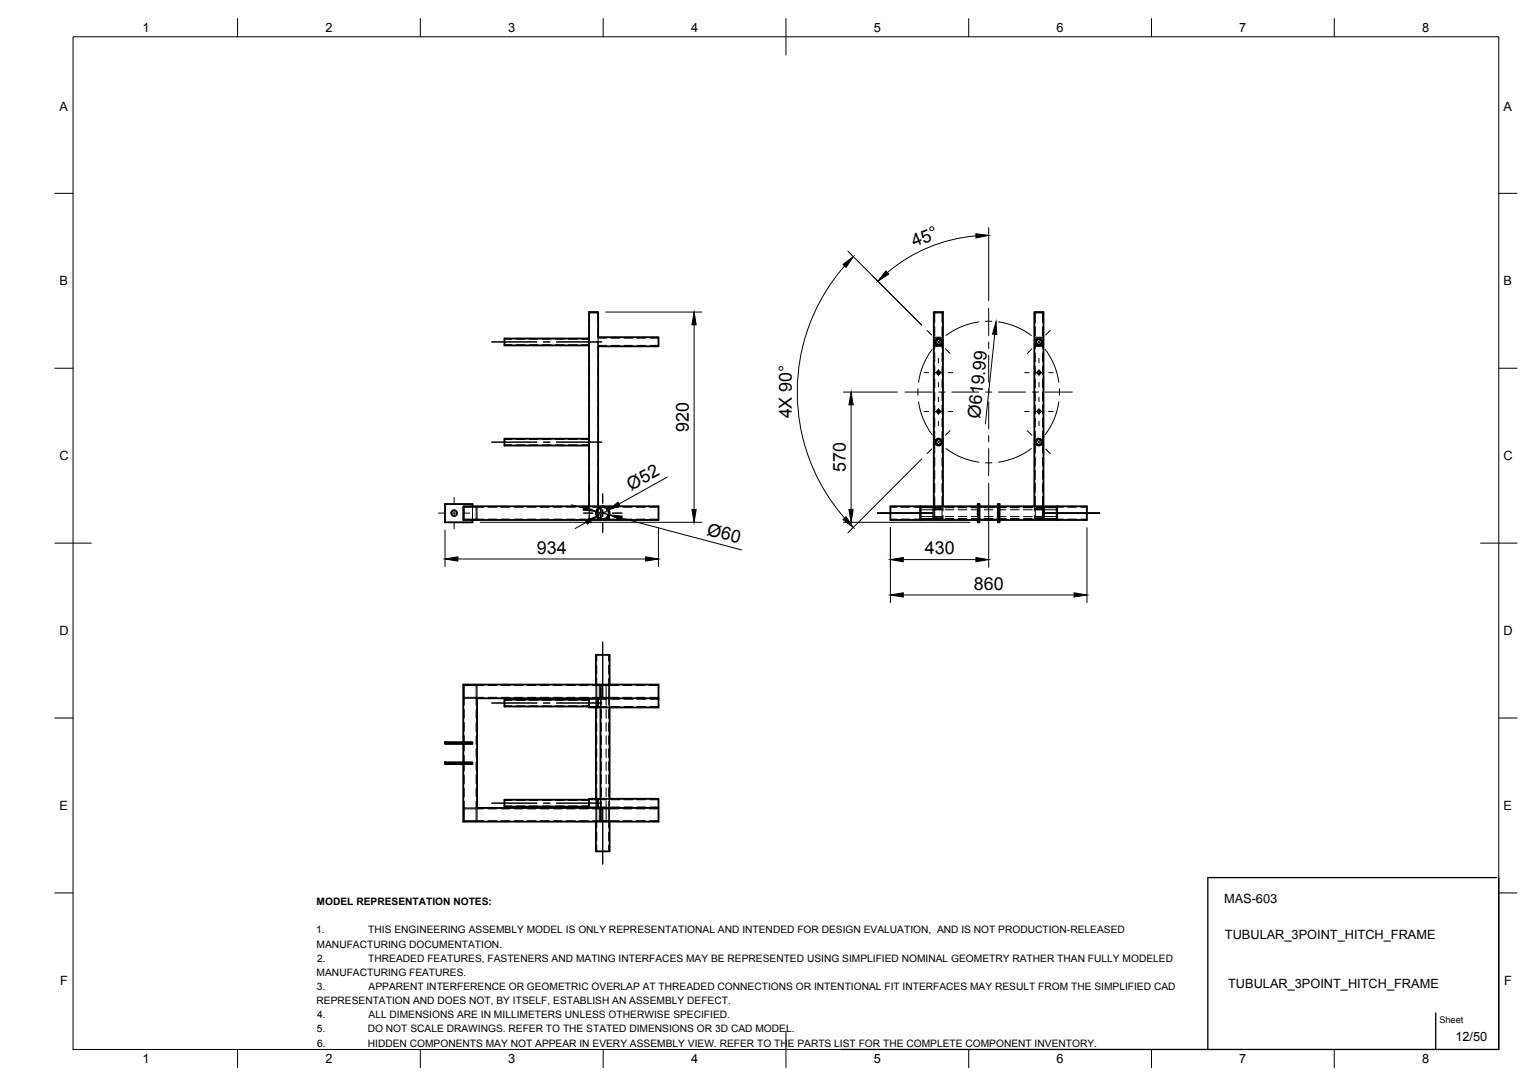
ISO-10303-21;
HEADER;
FILE_DESCRIPTION((''),'2;1');
FILE_NAME('TUBULAR_3POINT_HITCH_FRAME.step','2026-10-01T22:06:14-07:00',(''),(''),'','','');
FILE_SCHEMA (('AUTOMOTIVE_DESIGN { 1 0 10303 214 3 1 1 }'));
ENDSEC;
DATA;
#10=MECHANICAL_DESIGN_GEOMETRIC_PRESENTATION_REPRESENTATION('',(#986),#50440);
#49=ORIENTED_CLOSED_SHELL('',*,#28635,.F.) ;
#50=ORIENTED_CLOSED_SHELL('',*,#28636,.F.) ;
#51=ORIENTED_CLOSED_SHELL('',*,#28637,.F.) ;
#52=ORIENTED_CLOSED_SHELL('',*,#28638,.F.) ;
#53=ORIENTED_CLOSED_SHELL('',*,#28639,.F.) ;
#54=ORIENTED_CLOSED_SHELL('',*,#28640,.F.) ;
#55=ORIENTED_CLOSED_SHELL('',*,#28641,.F.) ;
#56=ORIENTED_CLOSED_SHELL('',*,#28642,.F.) ;
#57=ORIENTED_CLOSED_SHELL('',*,#28643,.F.) ;
#58=ORIENTED_CLOSED_SHELL('',*,#28644,.F.) ;
#59=ORIENTED_CLOSED_SHELL('',*,#28645,.F.) ;
#60=ORIENTED_CLOSED_SHELL('',*,#28646,.F.) ;
#61=ORIENTED_CLOSED_SHELL('',*,#28647,.F.) ;
#62=ORIENTED_CLOSED_SHELL('',*,#28648,.F.) ;
#63=ORIENTED_CLOSED_SHELL('',*,#28649,.F.) ;
#64=ORIENTED_CLOSED_SHELL('',*,#28650,.F.) ;
#65=ORIENTED_CLOSED_SHELL('',*,#28651,.F.) ;
#66=ORIENTED_CLOSED_SHELL('',*,#28652,.F.) ;
#67=ORIENTED_CLOSED_SHELL('',*,#28653,.F.) ;
#79=BREP_WITH_VOIDS('TUBULAR_3POINT_HITCH_FRAME',#28634,(#49,#50,#51,#52,
#53,#54,#55,#56,#57,#58,#59,#60,#61,#62,#63,#64,#65,#66,#67)) ;
#896=SHAPE_REPRESENTATION_RELATIONSHIP('SRR','None',#50627,#941) ;
#941=ADVANCED_BREP_SHAPE_REPRESENTATION('',(#79),#50396) ;
#986=STYLED_ITEM('',(#50883),#79) ;
#1234=FACE_BOUND('',#4462,.T.) ;
#1235=FACE_BOUND('',#4463,.T.) ;
#1236=FACE_BOUND('',#4465,.T.) ;
#1237=FACE_BOUND('',#4466,.T.) ;
#1238=FACE_BOUND('',#4476,.T.) ;
#1239=FACE_BOUND('',#4477,.T.) ;
#1240=FACE_BOUND('',#4479,.T.) ;
#1241=FACE_BOUND('',#4480,.T.) ;
#1242=FACE_BOUND('',#4488,.T.) ;
#1243=FACE_BOUND('',#4490,.T.) ;
#1244=FACE_BOUND('',#4491,.T.) ;
#1245=FACE_BOUND('',#4492,.T.) ;
#1246=FACE_BOUND('',#4493,.T.) ;
#1247=FACE_BOUND('',#4497,.T.) ;
#1248=FACE_BOUND('',#4504,.T.) ;
#1249=FACE_BOUND('',#4508,.T.) ;
#1250=FACE_BOUND('',#4509,.T.) ;
#1251=FACE_BOUND('',#4527,.T.) ;
#1252=FACE_BOUND('',#4536,.T.) ;
#1253=FACE_BOUND('',#4541,.T.) ;
#1254=FACE_BOUND('',#4550,.T.) ;
#1255=FACE_BOUND('',#4552,.T.) ;
#1256=FACE_BOUND('',#4564,.T.) ;
#1257=FACE_BOUND('',#4566,.T.) ;
#1258=FACE_BOUND('',#4569,.T.) ;
#1259=FACE_BOUND('',#4570,.T.) ;
#1260=FACE_BOUND('',#4574,.T.) ;
#1261=FACE_BOUND('',#4581,.T.) ;
#1262=FACE_BOUND('',#4585,.T.) ;
#1263=FACE_BOUND('',#4586,.T.) ;
#1264=FACE_BOUND('',#4587,.T.) ;
#1265=FACE_BOUND('',#4588,.T.) ;
#1266=FACE_BOUND('',#4590,.T.) ;
#1267=FACE_BOUND('',#4605,.T.) ;
#1268=FACE_BOUND('',#4609,.T.) ;
#1269=FACE_BOUND('',#4613,.T.) ;
#1729=PLANE('',#29943) ;
#1730=PLANE('',#29944) ;
#1731=PLANE('',#29945) ;
#1732=PLANE('',#29946) ;
#1733=PLANE('',#29947) ;
#1734=PLANE('',#29948) ;
#1735=PLANE('',#29949) ;
#1736=PLANE('',#29959) ;
#1737=PLANE('',#29960) ;
#1738=PLANE('',#29961) ;
#1739=PLANE('',#29962) ;
#1740=PLANE('',#29963) ;
#1741=PLANE('',#29964) ;
#1742=PLANE('',#29965) ;
#1743=PLANE('',#29978) ;
#1744=PLANE('',#29979) ;
#1745=PLANE('',#29986) ;
#1746=PLANE('',#29987) ;
#1747=PLANE('',#29988) ;
#1748=PLANE('',#29989) ;
#1749=PLANE('',#29990) ;
#1750=PLANE('',#29991) ;
#1751=PLANE('',#29992) ;
#1752=PLANE('',#29993) ;
#1753=PLANE('',#29994) ;
#1754=PLANE('',#29995) ;
#1755=PLANE('',#29996) ;
#1756=PLANE('',#29997) ;
#1757=PLANE('',#29998) ;
#1758=PLANE('',#30000) ;
#1759=PLANE('',#30001) ;
#1760=PLANE('',#30003) ;
#1761=PLANE('',#30004) ;
#1762=PLANE('',#30005) ;
#1763=PLANE('',#30007) ;
#1764=PLANE('',#30009) ;
#1765=PLANE('',#30010) ;
#1766=PLANE('',#30011) ;
#1767=PLANE('',#30012) ;
#1768=PLANE('',#30013) ;
#1769=PLANE('',#30014) ;
#1770=PLANE('',#30016) ;
#1771=PLANE('',#30018) ;
#1772=PLANE('',#30019) ;
#1773=PLANE('',#30021) ;
#1774=PLANE('',#30022) ;
#1775=PLANE('',#30023) ;
#1776=PLANE('',#30024) ;
#1777=PLANE('',#30025) ;
#1778=PLANE('',#30026) ;
#1779=PLANE('',#30027) ;
#1780=PLANE('',#30028) ;
#1781=PLANE('',#30029) ;
#1782=PLANE('',#30031) ;
#1783=PLANE('',#30033) ;
#1784=PLANE('',#30034) ;
#1785=PLANE('',#30035) ;
#1786=PLANE('',#30036) ;
#1787=PLANE('',#30038) ;
#1788=PLANE('',#30039) ;
#1789=PLANE('',#30040) ;
#1790=PLANE('',#30041) ;
#1791=PLANE('',#30042) ;
#1792=PLANE('',#30045) ;
#1793=PLANE('',#30052) ;
#1794=PLANE('',#30053) ;
#1795=PLANE('',#30054) ;
#1796=PLANE('',#30055) ;
#1797=PLANE('',#30056) ;
#1798=PLANE('',#30057) ;
#1799=PLANE('',#30058) ;
#1800=PLANE('',#30059) ;
#1801=PLANE('',#30060) ;
#1802=PLANE('',#30061) ;
#1803=PLANE('',#30062) ;
#1804=PLANE('',#30063) ;
#1805=PLANE('',#30064) ;
#1806=PLANE('',#30065) ;
#1807=PLANE('',#30066) ;
#1808=PLANE('',#30067) ;
#1809=PLANE('',#30068) ;
#1810=PLANE('',#30069) ;
#1811=PLANE('',#30071) ;
#1812=PLANE('',#30077) ;
#1813=PLANE('',#30079) ;
#1814=PLANE('',#30088) ;
#1815=PLANE('',#30089) ;
#1816=PLANE('',#30090) ;
#1817=PLANE('',#30091) ;
#1818=PLANE('',#30092) ;
#1819=PLANE('',#30093) ;
#1820=PLANE('',#30094) ;
#1821=PLANE('',#30095) ;
#1822=PLANE('',#30096) ;
#1823=PLANE('',#30097) ;
#1824=PLANE('',#30098) ;
#1825=PLANE('',#30099) ;
#1826=PLANE('',#30100) ;
#1827=PLANE('',#30101) ;
#1828=PLANE('',#30102) ;
#1829=PLANE('',#30103) ;
#1830=PLANE('',#30104) ;
#1831=PLANE('',#30105) ;
#1832=PLANE('',#30109) ;
#1833=PLANE('',#30110) ;
#1834=PLANE('',#30111) ;
#1835=PLANE('',#30112) ;
#1836=PLANE('',#30113) ;
#1837=PLANE('',#30114) ;
#1838=PLANE('',#30115) ;
#1839=PLANE('',#30117) ;
#1840=PLANE('',#30118) ;
#1841=PLANE('',#30120) ;
#1842=PLANE('',#30122) ;
#1843=PLANE('',#30124) ;
#1844=PLANE('',#30126) ;
#1845=PLANE('',#30128) ;
#1846=PLANE('',#30129) ;
#1847=PLANE('',#30130) ;
#1848=PLANE('',#30132) ;
#1849=PLANE('',#30135) ;
#1850=PLANE('',#30137) ;
#1851=PLANE('',#30138) ;
#1852=PLANE('',#30141) ;
#1853=PLANE('',#30142) ;
#1854=PLANE('',#30143) ;
#1855=PLANE('',#30144) ;
#1856=PLANE('',#30146) ;
#1857=PLANE('',#30149) ;
#1858=PLANE('',#30151) ;
#1859=PLANE('',#30154) ;
#1860=PLANE('',#30155) ;
#1861=PLANE('',#30156) ;
#1862=PLANE('',#30160) ;
#1863=PLANE('',#30161) ;
#1864=PLANE('',#30162) ;
#1865=PLANE('',#30163) ;
#1866=PLANE('',#30165) ;
#1867=PLANE('',#30168) ;
#1868=PLANE('',#30169) ;
#1869=PLANE('',#30170) ;
#1870=PLANE('',#30171) ;
#1871=PLANE('',#30173) ;
#1872=PLANE('',#30179) ;
#1873=PLANE('',#30180) ;
#1874=PLANE('',#30181) ;
#1875=PLANE('',#30182) ;
#1876=PLANE('',#30183) ;
#1877=PLANE('',#30185) ;
#1878=PLANE('',#30191) ;
#1879=PLANE('',#30192) ;
#1880=PLANE('',#30193) ;
#1881=PLANE('',#30194) ;
#1882=PLANE('',#30195) ;
#1883=PLANE('',#30199) ;
#1884=PLANE('',#30200) ;
#1885=PLANE('',#30201) ;
#1886=PLANE('',#30202) ;
#1887=PLANE('',#30203) ;
#1888=PLANE('',#30204) ;
#1889=PLANE('',#30205) ;
#1890=PLANE('',#30206) ;
#1891=PLANE('',#30207) ;
#1892=PLANE('',#30208) ;
#1893=PLANE('',#30209) ;
#1894=PLANE('',#30210) ;
#1895=PLANE('',#30211) ;
#1896=PLANE('',#30212) ;
#1897=PLANE('',#30213) ;
#1898=PLANE('',#30214) ;
#1899=PLANE('',#30215) ;
#1900=PLANE('',#30216) ;
#1901=PLANE('',#30217) ;
#1902=PLANE('',#30218) ;
#1903=PLANE('',#30219) ;
#1904=PLANE('',#30220) ;
#1905=PLANE('',#30221) ;
#1906=PLANE('',#30222) ;
#1907=PLANE('',#30223) ;
#1908=PLANE('',#30224) ;
#1909=PLANE('',#30225) ;
#1910=PLANE('',#30229) ;
#1911=PLANE('',#30230) ;
#1912=PLANE('',#30231) ;
#1913=PLANE('',#30232) ;
#1914=PLANE('',#30234) ;
#1915=PLANE('',#30241) ;
#1916=PLANE('',#30242) ;
#1917=PLANE('',#30243) ;
#1918=PLANE('',#30244) ;
#1919=PLANE('',#30245) ;
#2775=FACE_OUTER_BOUND('',#4451,.T.) ;
#2776=FACE_OUTER_BOUND('',#4452,.T.) ;
#2777=FACE_OUTER_BOUND('',#4453,.T.) ;
#2778=FACE_OUTER_BOUND('',#4454,.T.) ;
#2779=FACE_OUTER_BOUND('',#4455,.T.) ;
#2780=FACE_OUTER_BOUND('',#4456,.T.) ;
#2781=FACE_OUTER_BOUND('',#4457,.T.) ;
#2782=FACE_OUTER_BOUND('',#4458,.T.) ;
#2783=FACE_OUTER_BOUND('',#4459,.T.) ;
#2784=FACE_OUTER_BOUND('',#4460,.T.) ;
#2785=FACE_OUTER_BOUND('',#4461,.T.) ;
#2786=FACE_OUTER_BOUND('',#4464,.T.) ;
#2787=FACE_OUTER_BOUND('',#4467,.T.) ;
#2788=FACE_OUTER_BOUND('',#4468,.T.) ;
#2789=FACE_OUTER_BOUND('',#4469,.T.) ;
#2790=FACE_OUTER_BOUND('',#4470,.T.) ;
#2791=FACE_OUTER_BOUND('',#4471,.T.) ;
#2792=FACE_OUTER_BOUND('',#4472,.T.) ;
#2793=FACE_OUTER_BOUND('',#4473,.T.) ;
#2794=FACE_OUTER_BOUND('',#4474,.T.) ;
#2795=FACE_OUTER_BOUND('',#4475,.T.) ;
#2796=FACE_OUTER_BOUND('',#4478,.T.) ;
#2797=FACE_OUTER_BOUND('',#4481,.T.) ;
#2798=FACE_OUTER_BOUND('',#4482,.T.) ;
#2799=FACE_OUTER_BOUND('',#4483,.T.) ;
#2800=FACE_OUTER_BOUND('',#4484,.T.) ;
#2801=FACE_OUTER_BOUND('',#4485,.T.) ;
#2802=FACE_OUTER_BOUND('',#4486,.T.) ;
#2803=FACE_OUTER_BOUND('',#4487,.T.) ;
#2804=FACE_OUTER_BOUND('',#4489,.T.) ;
#2805=FACE_OUTER_BOUND('',#4494,.T.) ;
#2806=FACE_OUTER_BOUND('',#4495,.T.) ;
#2807=FACE_OUTER_BOUND('',#4496,.T.) ;
#2808=FACE_OUTER_BOUND('',#4498,.T.) ;
#2809=FACE_OUTER_BOUND('',#4499,.T.) ;
#2810=FACE_OUTER_BOUND('',#4500,.T.) ;
#2811=FACE_OUTER_BOUND('',#4501,.T.) ;
#2812=FACE_OUTER_BOUND('',#4502,.T.) ;
#2813=FACE_OUTER_BOUND('',#4503,.T.) ;
#2814=FACE_OUTER_BOUND('',#4505,.T.) ;
#2815=FACE_OUTER_BOUND('',#4506,.T.) ;
#2816=FACE_OUTER_BOUND('',#4507,.T.) ;
#2817=FACE_OUTER_BOUND('',#4510,.T.) ;
#2818=FACE_OUTER_BOUND('',#4511,.T.) ;
#2819=FACE_OUTER_BOUND('',#4512,.T.) ;
#2820=FACE_OUTER_BOUND('',#4513,.T.) ;
#2821=FACE_OUTER_BOUND('',#4514,.T.) ;
#2822=FACE_OUTER_BOUND('',#4515,.T.) ;
#2823=FACE_OUTER_BOUND('',#4516,.T.) ;
#2824=FACE_OUTER_BOUND('',#4517,.T.) ;
#2825=FACE_OUTER_BOUND('',#4518,.T.) ;
#2826=FACE_OUTER_BOUND('',#4519,.T.) ;
#2827=FACE_OUTER_BOUND('',#4520,.T.) ;
#2828=FACE_OUTER_BOUND('',#4521,.T.) ;
#2829=FACE_OUTER_BOUND('',#4522,.T.) ;
#2830=FACE_OUTER_BOUND('',#4523,.T.) ;
#2831=FACE_OUTER_BOUND('',#4524,.T.) ;
#2832=FACE_OUTER_BOUND('',#4525,.T.) ;
#2833=FACE_OUTER_BOUND('',#4526,.T.) ;
#2834=FACE_OUTER_BOUND('',#4528,.T.) ;
#2835=FACE_OUTER_BOUND('',#4529,.T.) ;
#2836=FACE_OUTER_BOUND('',#4530,.T.) ;
#2837=FACE_OUTER_BOUND('',#4531,.T.) ;
#2838=FACE_OUTER_BOUND('',#4532,.T.) ;
#2839=FACE_OUTER_BOUND('',#4533,.T.) ;
#2840=FACE_OUTER_BOUND('',#4534,.T.) ;
#2841=FACE_OUTER_BOUND('',#4535,.T.) ;
#2842=FACE_OUTER_BOUND('',#4537,.T.) ;
#2843=FACE_OUTER_BOUND('',#4538,.T.) ;
#2844=FACE_OUTER_BOUND('',#4539,.T.) ;
#2845=FACE_OUTER_BOUND('',#4540,.T.) ;
#2846=FACE_OUTER_BOUND('',#4542,.T.) ;
#2847=FACE_OUTER_BOUND('',#4543,.T.) ;
#2848=FACE_OUTER_BOUND('',#4544,.T.) ;
#2849=FACE_OUTER_BOUND('',#4545,.T.) ;
#2850=FACE_OUTER_BOUND('',#4546,.T.) ;
#2851=FACE_OUTER_BOUND('',#4547,.T.) ;
#2852=FACE_OUTER_BOUND('',#4548,.T.) ;
#2853=FACE_OUTER_BOUND('',#4549,.T.) ;
#2854=FACE_OUTER_BOUND('',#4551,.T.) ;
#2855=FACE_OUTER_BOUND('',#4553,.T.) ;
#2856=FACE_OUTER_BOUND('',#4554,.T.) ;
#2857=FACE_OUTER_BOUND('',#4555,.T.) ;
#2858=FACE_OUTER_BOUND('',#4556,.T.) ;
#2859=FACE_OUTER_BOUND('',#4557,.T.) ;
#2860=FACE_OUTER_BOUND('',#4558,.T.) ;
#2861=FACE_OUTER_BOUND('',#4559,.T.) ;
#2862=FACE_OUTER_BOUND('',#4560,.T.) ;
#2863=FACE_OUTER_BOUND('',#4561,.T.) ;
#2864=FACE_OUTER_BOUND('',#4562,.T.) ;
#2865=FACE_OUTER_BOUND('',#4563,.T.) ;
#2866=FACE_OUTER_BOUND('',#4565,.T.) ;
#2867=FACE_OUTER_BOUND('',#4567,.T.) ;
#2868=FACE_OUTER_BOUND('',#4568,.T.) ;
#2869=FACE_OUTER_BOUND('',#4571,.T.) ;
#2870=FACE_OUTER_BOUND('',#4572,.T.) ;
#2871=FACE_OUTER_BOUND('',#4573,.T.) ;
#2872=FACE_OUTER_BOUND('',#4575,.T.) ;
#2873=FACE_OUTER_BOUND('',#4576,.T.) ;
#2874=FACE_OUTER_BOUND('',#4577,.T.) ;
#2875=FACE_OUTER_BOUND('',#4578,.T.) ;
#2876=FACE_OUTER_BOUND('',#4579,.T.) ;
#2877=FACE_OUTER_BOUND('',#4580,.T.) ;
#2878=FACE_OUTER_BOUND('',#4582,.T.) ;
#2879=FACE_OUTER_BOUND('',#4583,.T.) ;
#2880=FACE_OUTER_BOUND('',#4584,.T.) ;
#2881=FACE_OUTER_BOUND('',#4589,.T.) ;
#2882=FACE_OUTER_BOUND('',#4591,.T.) ;
#2883=FACE_OUTER_BOUND('',#4592,.T.) ;
#2884=FACE_OUTER_BOUND('',#4593,.T.) ;
#2885=FACE_OUTER_BOUND('',#4594,.T.) ;
#2886=FACE_OUTER_BOUND('',#4595,.T.) ;
#2887=FACE_OUTER_BOUND('',#4596,.T.) ;
#2888=FACE_OUTER_BOUND('',#4597,.T.) ;
#2889=FACE_OUTER_BOUND('',#4598,.T.) ;
#2890=FACE_OUTER_BOUND('',#4599,.T.) ;
#2891=FACE_OUTER_BOUND('',#4600,.T.) ;
#2892=FACE_OUTER_BOUND('',#4601,.T.) ;
#2893=FACE_OUTER_BOUND('',#4602,.T.) ;
#2894=FACE_OUTER_BOUND('',#4603,.T.) ;
#2895=FACE_OUTER_BOUND('',#4604,.T.) ;
#2896=FACE_OUTER_BOUND('',#4606,.T.) ;
#2897=FACE_OUTER_BOUND('',#4607,.T.) ;
#2898=FACE_OUTER_BOUND('',#4608,.T.) ;
#2899=FACE_OUTER_BOUND('',#4610,.T.) ;
#2900=FACE_OUTER_BOUND('',#4611,.T.) ;
#2901=FACE_OUTER_BOUND('',#4612,.T.) ;
#2902=FACE_OUTER_BOUND('',#4614,.T.) ;
#2903=FACE_OUTER_BOUND('',#4615,.T.) ;
#2904=FACE_OUTER_BOUND('',#4616,.T.) ;
#2905=FACE_OUTER_BOUND('',#4617,.T.) ;
#2906=FACE_OUTER_BOUND('',#4618,.T.) ;
#2907=FACE_OUTER_BOUND('',#4619,.T.) ;
#2908=FACE_OUTER_BOUND('',#4620,.T.) ;
#2909=FACE_OUTER_BOUND('',#4621,.T.) ;
#2910=FACE_OUTER_BOUND('',#4622,.T.) ;
#2911=FACE_OUTER_BOUND('',#4623,.T.) ;
#2912=FACE_OUTER_BOUND('',#4624,.T.) ;
#2913=FACE_OUTER_BOUND('',#4625,.T.) ;
#2914=FACE_OUTER_BOUND('',#4626,.T.) ;
#2915=FACE_OUTER_BOUND('',#4627,.T.) ;
#2916=FACE_OUTER_BOUND('',#4628,.T.) ;
#2917=FACE_OUTER_BOUND('',#4629,.T.) ;
#2918=FACE_OUTER_BOUND('',#4630,.T.) ;
#2919=FACE_OUTER_BOUND('',#4631,.T.) ;
#2920=FACE_OUTER_BOUND('',#4632,.T.) ;
#2921=FACE_OUTER_BOUND('',#4633,.T.) ;
#2922=FACE_OUTER_BOUND('',#4634,.T.) ;
#2923=FACE_OUTER_BOUND('',#4635,.T.) ;
#2924=FACE_OUTER_BOUND('',#4636,.T.) ;
#2925=FACE_OUTER_BOUND('',#4637,.T.) ;
#2926=FACE_OUTER_BOUND('',#4638,.T.) ;
#2927=FACE_OUTER_BOUND('',#4639,.T.) ;
#2928=FACE_OUTER_BOUND('',#4640,.T.) ;
#2929=FACE_OUTER_BOUND('',#4641,.T.) ;
#2930=FACE_OUTER_BOUND('',#4642,.T.) ;
#2931=FACE_OUTER_BOUND('',#4643,.T.) ;
#2932=FACE_OUTER_BOUND('',#4644,.T.) ;
#2933=FACE_OUTER_BOUND('',#4645,.T.) ;
#2934=FACE_OUTER_BOUND('',#4646,.T.) ;
#2935=FACE_OUTER_BOUND('',#4647,.T.) ;
#2936=FACE_OUTER_BOUND('',#4648,.T.) ;
#2937=FACE_OUTER_BOUND('',#4649,.T.) ;
#2938=FACE_OUTER_BOUND('',#4650,.T.) ;
#2939=FACE_OUTER_BOUND('',#4651,.T.) ;
#2940=FACE_OUTER_BOUND('',#4652,.T.) ;
#2941=FACE_OUTER_BOUND('',#4653,.T.) ;
#2942=FACE_OUTER_BOUND('',#4654,.T.) ;
#2943=FACE_OUTER_BOUND('',#4655,.T.) ;
#2944=FACE_OUTER_BOUND('',#4656,.T.) ;
#2945=FACE_OUTER_BOUND('',#4657,.T.) ;
#2946=FACE_OUTER_BOUND('',#4658,.T.) ;
#2947=FACE_OUTER_BOUND('',#4659,.T.) ;
#2948=FACE_OUTER_BOUND('',#4660,.T.) ;
#2949=FACE_OUTER_BOUND('',#4661,.T.) ;
#2950=FACE_OUTER_BOUND('',#4662,.T.) ;
#2951=FACE_OUTER_BOUND('',#4663,.T.) ;
#2952=FACE_OUTER_BOUND('',#4664,.T.) ;
#2953=FACE_OUTER_BOUND('',#4665,.T.) ;
#2954=FACE_OUTER_BOUND('',#4666,.T.) ;
#2955=FACE_OUTER_BOUND('',#4667,.T.) ;
#2956=FACE_OUTER_BOUND('',#4668,.T.) ;
#2957=FACE_OUTER_BOUND('',#4669,.T.) ;
#2958=FACE_OUTER_BOUND('',#4670,.T.) ;
#2959=FACE_OUTER_BOUND('',#4671,.T.) ;
#2960=FACE_OUTER_BOUND('',#4672,.T.) ;
#2961=FACE_OUTER_BOUND('',#4673,.T.) ;
#2962=FACE_OUTER_BOUND('',#4674,.T.) ;
#2963=FACE_OUTER_BOUND('',#4675,.T.) ;
#2964=FACE_OUTER_BOUND('',#4676,.T.) ;
#2965=FACE_OUTER_BOUND('',#4677,.T.) ;
#2966=FACE_OUTER_BOUND('',#4678,.T.) ;
#2967=FACE_OUTER_BOUND('',#4679,.T.) ;
#2968=FACE_OUTER_BOUND('',#4680,.T.) ;
#2969=FACE_OUTER_BOUND('',#4681,.T.) ;
#2970=FACE_OUTER_BOUND('',#4682,.T.) ;
#2971=FACE_OUTER_BOUND('',#4683,.T.) ;
#2972=FACE_OUTER_BOUND('',#4684,.T.) ;
#2973=FACE_OUTER_BOUND('',#4685,.T.) ;
#2974=FACE_OUTER_BOUND('',#4686,.T.) ;
#2975=FACE_OUTER_BOUND('',#4687,.T.) ;
#2976=FACE_OUTER_BOUND('',#4688,.T.) ;
#2977=FACE_OUTER_BOUND('',#4689,.T.) ;
#2978=FACE_OUTER_BOUND('',#4690,.T.) ;
#2979=FACE_OUTER_BOUND('',#4691,.T.) ;
#2980=FACE_OUTER_BOUND('',#4692,.T.) ;
#2981=FACE_OUTER_BOUND('',#4693,.T.) ;
#2982=FACE_OUTER_BOUND('',#4694,.T.) ;
#2983=FACE_OUTER_BOUND('',#4695,.T.) ;
#2984=FACE_OUTER_BOUND('',#4696,.T.) ;
#2985=FACE_OUTER_BOUND('',#4697,.T.) ;
#2986=FACE_OUTER_BOUND('',#4698,.T.) ;
#2987=FACE_OUTER_BOUND('',#4699,.T.) ;
#2988=FACE_OUTER_BOUND('',#4700,.T.) ;
#2989=FACE_OUTER_BOUND('',#4701,.T.) ;
#2990=FACE_OUTER_BOUND('',#4702,.T.) ;
#2991=FACE_OUTER_BOUND('',#4703,.T.) ;
#2992=FACE_OUTER_BOUND('',#4704,.T.) ;
#2993=FACE_OUTER_BOUND('',#4705,.T.) ;
#2994=FACE_OUTER_BOUND('',#4706,.T.) ;
#2995=FACE_OUTER_BOUND('',#4707,.T.) ;
#2996=FACE_OUTER_BOUND('',#4708,.T.) ;
#2997=FACE_OUTER_BOUND('',#4709,.T.) ;
#2998=FACE_OUTER_BOUND('',#4710,.T.) ;
#2999=FACE_OUTER_BOUND('',#4711,.T.) ;
#3000=FACE_OUTER_BOUND('',#4712,.T.) ;
#3001=FACE_OUTER_BOUND('',#4713,.T.) ;
#3002=FACE_OUTER_BOUND('',#4714,.T.) ;
#3003=FACE_OUTER_BOUND('',#4715,.T.) ;
#3004=FACE_OUTER_BOUND('',#4716,.T.) ;
#3005=FACE_OUTER_BOUND('',#4717,.T.) ;
#3006=FACE_OUTER_BOUND('',#4718,.T.) ;
#4451=EDGE_LOOP('',(#21063,#21064,#21065,#21066)) ;
#4452=EDGE_LOOP('',(#21067,#21068,#21069,#21070)) ;
#4453=EDGE_LOOP('',(#21071,#21072,#21073,#21074)) ;
#4454=EDGE_LOOP('',(#21075,#21076,#21077,#21078)) ;
#4455=EDGE_LOOP('',(#21079,#21080,#21081,#21082)) ;
#4456=EDGE_LOOP('',(#21083,#21084,#21085,#21086)) ;
#4457=EDGE_LOOP('',(#21087,#21088,#21089,#21090)) ;
#4458=EDGE_LOOP('',(#21091,#21092,#21093,#21094)) ;
#4459=EDGE_LOOP('',(#21095,#21096,#21097,#21098,#21099,#21100)) ;
#4460=EDGE_LOOP('',(#21101,#21102,#21103,#21104)) ;
#4461=EDGE_LOOP('',(#21105,#21106,#21107,#21108)) ;
#4462=EDGE_LOOP('',(#21109)) ;
#4463=EDGE_LOOP('',(#21110)) ;
#4464=EDGE_LOOP('',(#21111,#21112,#21113,#21114)) ;
#4465=EDGE_LOOP('',(#21115)) ;
#4466=EDGE_LOOP('',(#21116)) ;
#4467=EDGE_LOOP('',(#21117,#21118,#21119,#21120)) ;
#4468=EDGE_LOOP('',(#21121,#21122,#21123,#21124,#21125,#21126)) ;
#4469=EDGE_LOOP('',(#21127,#21128,#21129,#21130)) ;
#4470=EDGE_LOOP('',(#21131,#21132,#21133,#21134)) ;
#4471=EDGE_LOOP('',(#21135,#21136,#21137,#21138)) ;
#4472=EDGE_LOOP('',(#21139,#21140,#21141,#21142)) ;
#4473=EDGE_LOOP('',(#21143,#21144,#21145,#21146,#21147,#21148)) ;
#4474=EDGE_LOOP('',(#21149,#21150,#21151,#21152)) ;
#4475=EDGE_LOOP('',(#21153,#21154,#21155,#21156)) ;
#4476=EDGE_LOOP('',(#21157)) ;
#4477=EDGE_LOOP('',(#21158)) ;
#4478=EDGE_LOOP('',(#21159,#21160,#21161,#21162)) ;
#4479=EDGE_LOOP('',(#21163)) ;
#4480=EDGE_LOOP('',(#21164)) ;
#4481=EDGE_LOOP('',(#21165,#21166,#21167,#21168)) ;
#4482=EDGE_LOOP('',(#21169,#21170,#21171,#21172,#21173,#21174)) ;
#4483=EDGE_LOOP('',(#21175,#21176,#21177,#21178)) ;
#4484=EDGE_LOOP('',(#21179,#21180,#21181,#21182)) ;
#4485=EDGE_LOOP('',(#21183,#21184,#21185,#21186)) ;
#4486=EDGE_LOOP('',(#21187,#21188,#21189,#21190)) ;
#4487=EDGE_LOOP('',(#21191)) ;
#4488=EDGE_LOOP('',(#21192)) ;
#4489=EDGE_LOOP('',(#21193,#21194,#21195,#21196,#21197)) ;
#4490=EDGE_LOOP('',(#21198)) ;
#4491=EDGE_LOOP('',(#21199)) ;
#4492=EDGE_LOOP('',(#21200)) ;
#4493=EDGE_LOOP('',(#21201)) ;
#4494=EDGE_LOOP('',(#21202,#21203,#21204,#21205)) ;
#4495=EDGE_LOOP('',(#21206,#21207,#21208,#21209)) ;
#4496=EDGE_LOOP('',(#21210)) ;
#4497=EDGE_LOOP('',(#21211)) ;
#4498=EDGE_LOOP('',(#21212)) ;
#4499=EDGE_LOOP('',(#21213,#21214,#21215,#21216)) ;
#4500=EDGE_LOOP('',(#21217,#21218,#21219,#21220)) ;
#4501=EDGE_LOOP('',(#21221,#21222,#21223,#21224)) ;
#4502=EDGE_LOOP('',(#21225,#21226,#21227,#21228)) ;
#4503=EDGE_LOOP('',(#21229,#21230,#21231,#21232)) ;
#4504=EDGE_LOOP('',(#21233,#21234,#21235,#21236)) ;
#4505=EDGE_LOOP('',(#21237,#21238,#21239,#21240)) ;
#4506=EDGE_LOOP('',(#21241,#21242,#21243,#21244)) ;
#4507=EDGE_LOOP('',(#21245,#21246,#21247,#21248,#21249)) ;
#4508=EDGE_LOOP('',(#21250)) ;
#4509=EDGE_LOOP('',(#21251)) ;
#4510=EDGE_LOOP('',(#21252,#21253,#21254,#21255)) ;
#4511=EDGE_LOOP('',(#21256,#21257,#21258,#21259)) ;
#4512=EDGE_LOOP('',(#21260)) ;
#4513=EDGE_LOOP('',(#21261,#21262,#21263,#21264)) ;
#4514=EDGE_LOOP('',(#21265,#21266,#21267,#21268,#21269,#21270,#21271,#21272,
#21273,#21274)) ;
#4515=EDGE_LOOP('',(#21275,#21276,#21277,#21278,#21279,#21280,#21281,#21282)) ;
#4516=EDGE_LOOP('',(#21283,#21284,#21285,#21286)) ;
#4517=EDGE_LOOP('',(#21287,#21288,#21289,#21290)) ;
#4518=EDGE_LOOP('',(#21291,#21292,#21293,#21294)) ;
#4519=EDGE_LOOP('',(#21295,#21296,#21297,#21298)) ;
#4520=EDGE_LOOP('',(#21299,#21300,#21301,#21302)) ;
#4521=EDGE_LOOP('',(#21303,#21304,#21305,#21306)) ;
#4522=EDGE_LOOP('',(#21307,#21308,#21309,#21310)) ;
#4523=EDGE_LOOP('',(#21311,#21312,#21313,#21314)) ;
#4524=EDGE_LOOP('',(#21315,#21316,#21317,#21318)) ;
#4525=EDGE_LOOP('',(#21319,#21320,#21321,#21322)) ;
#4526=EDGE_LOOP('',(#21323,#21324,#21325,#21326,#21327,#21328,#21329,#21330,
#21331,#21332,#21333,#21334,#21335,#21336,#21337,#21338,#21339,#21340)) ;
#4527=EDGE_LOOP('',(#21341,#21342,#21343,#21344,#21345,#21346,#21347,#21348,
#21349,#21350,#21351,#21352)) ;
#4528=EDGE_LOOP('',(#21353,#21354,#21355,#21356)) ;
#4529=EDGE_LOOP('',(#21357,#21358,#21359,#21360)) ;
#4530=EDGE_LOOP('',(#21361,#21362,#21363,#21364)) ;
#4531=EDGE_LOOP('',(#21365,#21366,#21367,#21368)) ;
#4532=EDGE_LOOP('',(#21369,#21370,#21371,#21372)) ;
#4533=EDGE_LOOP('',(#21373,#21374,#21375,#21376)) ;
#4534=EDGE_LOOP('',(#21377,#21378,#21379,#21380)) ;
#4535=EDGE_LOOP('',(#21381,#21382,#21383,#21384)) ;
#4536=EDGE_LOOP('',(#21385,#21386,#21387,#21388)) ;
#4537=EDGE_LOOP('',(#21389,#21390,#21391,#21392)) ;
#4538=EDGE_LOOP('',(#21393)) ;
#4539=EDGE_LOOP('',(#21394)) ;
#4540=EDGE_LOOP('',(#21395,#21396,#21397,#21398)) ;
#4541=EDGE_LOOP('',(#21399,#21400,#21401,#21402)) ;
#4542=EDGE_LOOP('',(#21403,#21404,#21405,#21406)) ;
#4543=EDGE_LOOP('',(#21407,#21408,#21409,#21410)) ;
#4544=EDGE_LOOP('',(#21411,#21412,#21413,#21414)) ;
#4545=EDGE_LOOP('',(#21415,#21416,#21417,#21418)) ;
#4546=EDGE_LOOP('',(#21419,#21420,#21421,#21422)) ;
#4547=EDGE_LOOP('',(#21423,#21424,#21425,#21426)) ;
#4548=EDGE_LOOP('',(#21427,#21428,#21429,#21430)) ;
#4549=EDGE_LOOP('',(#21431)) ;
#4550=EDGE_LOOP('',(#21432)) ;
#4551=EDGE_LOOP('',(#21433)) ;
#4552=EDGE_LOOP('',(#21434)) ;
#4553=EDGE_LOOP('',(#21435,#21436,#21437,#21438,#21439)) ;
#4554=EDGE_LOOP('',(#21440,#21441,#21442,#21443,#21444)) ;
#4555=EDGE_LOOP('',(#21445,#21446,#21447,#21448)) ;
#4556=EDGE_LOOP('',(#21449,#21450,#21451,#21452)) ;
#4557=EDGE_LOOP('',(#21453,#21454,#21455,#21456)) ;
#4558=EDGE_LOOP('',(#21457,#21458,#21459,#21460)) ;
#4559=EDGE_LOOP('',(#21461,#21462,#21463,#21464)) ;
#4560=EDGE_LOOP('',(#21465,#21466,#21467,#21468)) ;
#4561=EDGE_LOOP('',(#21469,#21470,#21471,#21472)) ;
#4562=EDGE_LOOP('',(#21473,#21474,#21475,#21476)) ;
#4563=EDGE_LOOP('',(#21477,#21478,#21479,#21480,#21481,#21482,#21483,#21484)) ;
#4564=EDGE_LOOP('',(#21485)) ;
#4565=EDGE_LOOP('',(#21486,#21487,#21488,#21489,#21490,#21491,#21492,#21493)) ;
#4566=EDGE_LOOP('',(#21494)) ;
#4567=EDGE_LOOP('',(#21495,#21496,#21497,#21498)) ;
#4568=EDGE_LOOP('',(#21499,#21500,#21501,#21502,#21503)) ;
#4569=EDGE_LOOP('',(#21504)) ;
#4570=EDGE_LOOP('',(#21505)) ;
#4571=EDGE_LOOP('',(#21506,#21507,#21508,#21509)) ;
#4572=EDGE_LOOP('',(#21510,#21511,#21512,#21513)) ;
#4573=EDGE_LOOP('',(#21514,#21515,#21516,#21517)) ;
#4574=EDGE_LOOP('',(#21518,#21519,#21520,#21521)) ;
#4575=EDGE_LOOP('',(#21522,#21523,#21524,#21525)) ;
#4576=EDGE_LOOP('',(#21526,#21527,#21528,#21529)) ;
#4577=EDGE_LOOP('',(#21530,#21531,#21532,#21533)) ;
#4578=EDGE_LOOP('',(#21534,#21535,#21536,#21537)) ;
#4579=EDGE_LOOP('',(#21538)) ;
#4580=EDGE_LOOP('',(#21539)) ;
#4581=EDGE_LOOP('',(#21540)) ;
#4582=EDGE_LOOP('',(#21541,#21542,#21543,#21544)) ;
#4583=EDGE_LOOP('',(#21545,#21546,#21547,#21548)) ;
#4584=EDGE_LOOP('',(#21549,#21550,#21551,#21552,#21553)) ;
#4585=EDGE_LOOP('',(#21554)) ;
#4586=EDGE_LOOP('',(#21555)) ;
#4587=EDGE_LOOP('',(#21556)) ;
#4588=EDGE_LOOP('',(#21557)) ;
#4589=EDGE_LOOP('',(#21558)) ;
#4590=EDGE_LOOP('',(#21559)) ;
#4591=EDGE_LOOP('',(#21560,#21561,#21562,#21563)) ;
#4592=EDGE_LOOP('',(#21564,#21565,#21566,#21567)) ;
#4593=EDGE_LOOP('',(#21568,#21569,#21570,#21571,#21572,#21573,#21574,#21575,
#21576,#21577,#21578,#21579)) ;
#4594=EDGE_LOOP('',(#21580,#21581,#21582,#21583)) ;
#4595=EDGE_LOOP('',(#21584,#21585,#21586,#21587)) ;
#4596=EDGE_LOOP('',(#21588,#21589,#21590,#21591)) ;
#4597=EDGE_LOOP('',(#21592,#21593,#21594,#21595)) ;
#4598=EDGE_LOOP('',(#21596,#21597,#21598,#21599,#21600,#21601,#21602,#21603,
#21604,#21605)) ;
#4599=EDGE_LOOP('',(#21606)) ;
#4600=EDGE_LOOP('',(#21607,#21608,#21609,#21610)) ;
#4601=EDGE_LOOP('',(#21611,#21612,#21613,#21614)) ;
#4602=EDGE_LOOP('',(#21615,#21616,#21617,#21618,#21619,#21620,#21621,#21622)) ;
#4603=EDGE_LOOP('',(#21623,#21624,#21625,#21626)) ;
#4604=EDGE_LOOP('',(#21627,#21628,#21629,#21630,#21631,#21632,#21633,#21634,
#21635,#21636,#21637,#21638,#21639,#21640,#21641,#21642,#21643,#21644)) ;
#4605=EDGE_LOOP('',(#21645,#21646,#21647,#21648,#21649,#21650,#21651,#21652)) ;
#4606=EDGE_LOOP('',(#21653,#21654,#21655,#21656)) ;
#4607=EDGE_LOOP('',(#21657,#21658,#21659,#21660)) ;
#4608=EDGE_LOOP('',(#21661,#21662,#21663,#21664,#21665,#21666,#21667,#21668)) ;
#4609=EDGE_LOOP('',(#21669)) ;
#4610=EDGE_LOOP('',(#21670,#21671,#21672,#21673)) ;
#4611=EDGE_LOOP('',(#21674,#21675,#21676,#21677)) ;
#4612=EDGE_LOOP('',(#21678,#21679,#21680,#21681,#21682,#21683,#21684,#21685)) ;
#4613=EDGE_LOOP('',(#21686)) ;
#4614=EDGE_LOOP('',(#21687,#21688,#21689,#21690)) ;
#4615=EDGE_LOOP('',(#21691,#21692,#21693,#21694)) ;
#4616=EDGE_LOOP('',(#21695,#21696,#21697,#21698)) ;
#4617=EDGE_LOOP('',(#21699,#21700,#21701,#21702)) ;
#4618=EDGE_LOOP('',(#21703,#21704,#21705,#21706)) ;
#4619=EDGE_LOOP('',(#21707,#21708,#21709,#21710)) ;
#4620=EDGE_LOOP('',(#21711,#21712,#21713,#21714)) ;
#4621=EDGE_LOOP('',(#21715,#21716,#21717,#21718)) ;
#4622=EDGE_LOOP('',(#21719,#21720,#21721,#21722)) ;
#4623=EDGE_LOOP('',(#21723,#21724,#21725,#21726)) ;
#4624=EDGE_LOOP('',(#21727,#21728,#21729,#21730)) ;
#4625=EDGE_LOOP('',(#21731,#21732,#21733,#21734)) ;
#4626=EDGE_LOOP('',(#21735,#21736,#21737,#21738)) ;
#4627=EDGE_LOOP('',(#21739,#21740)) ;
#4628=EDGE_LOOP('',(#21741,#21742)) ;
#4629=EDGE_LOOP('',(#21743,#21744,#21745,#21746)) ;
#4630=EDGE_LOOP('',(#21747,#21748,#21749,#21750)) ;
#4631=EDGE_LOOP('',(#21751,#21752,#21753,#21754)) ;
#4632=EDGE_LOOP('',(#21755,#21756,#21757,#21758)) ;
#4633=EDGE_LOOP('',(#21759,#21760,#21761)) ;
#4634=EDGE_LOOP('',(#21762,#21763,#21764)) ;
#4635=EDGE_LOOP('',(#21765,#21766,#21767,#21768)) ;
#4636=EDGE_LOOP('',(#21769,#21770,#21771)) ;
#4637=EDGE_LOOP('',(#21772,#21773,#21774,#21775)) ;
#4638=EDGE_LOOP('',(#21776,#21777,#21778)) ;
#4639=EDGE_LOOP('',(#21779,#21780,#21781,#21782)) ;
#4640=EDGE_LOOP('',(#21783,#21784,#21785,#21786)) ;
#4641=EDGE_LOOP('',(#21787,#21788,#21789,#21790)) ;
#4642=EDGE_LOOP('',(#21791,#21792,#21793,#21794)) ;
#4643=EDGE_LOOP('',(#21795,#21796,#21797)) ;
#4644=EDGE_LOOP('',(#21798,#21799,#21800)) ;
#4645=EDGE_LOOP('',(#21801,#21802,#21803,#21804)) ;
#4646=EDGE_LOOP('',(#21805,#21806,#21807)) ;
#4647=EDGE_LOOP('',(#21808,#21809,#21810)) ;
#4648=EDGE_LOOP('',(#21811,#21812,#21813,#21814)) ;
#4649=EDGE_LOOP('',(#21815,#21816,#21817,#21818)) ;
#4650=EDGE_LOOP('',(#21819,#21820,#21821,#21822)) ;
#4651=EDGE_LOOP('',(#21823,#21824,#21825,#21826)) ;
#4652=EDGE_LOOP('',(#21827,#21828,#21829,#21830)) ;
#4653=EDGE_LOOP('',(#21831,#21832,#21833)) ;
#4654=EDGE_LOOP('',(#21834,#21835,#21836,#21837)) ;
#4655=EDGE_LOOP('',(#21838,#21839,#21840)) ;
#4656=EDGE_LOOP('',(#21841,#21842,#21843)) ;
#4657=EDGE_LOOP('',(#21844,#21845,#21846)) ;
#4658=EDGE_LOOP('',(#21847,#21848,#21849,#21850)) ;
#4659=EDGE_LOOP('',(#21851,#21852,#21853,#21854)) ;
#4660=EDGE_LOOP('',(#21855,#21856,#21857,#21858)) ;
#4661=EDGE_LOOP('',(#21859,#21860,#21861,#21862)) ;
#4662=EDGE_LOOP('',(#21863,#21864)) ;
#4663=EDGE_LOOP('',(#21865,#21866)) ;
#4664=EDGE_LOOP('',(#21867,#21868,#21869,#21870)) ;
#4665=EDGE_LOOP('',(#21871,#21872,#21873,#21874)) ;
#4666=EDGE_LOOP('',(#21875,#21876)) ;
#4667=EDGE_LOOP('',(#21877,#21878)) ;
#4668=EDGE_LOOP('',(#21879,#21880,#21881,#21882)) ;
#4669=EDGE_LOOP('',(#21883,#21884,#21885,#21886)) ;
#4670=EDGE_LOOP('',(#21887,#21888)) ;
#4671=EDGE_LOOP('',(#21889,#21890)) ;
#4672=EDGE_LOOP('',(#21891,#21892,#21893,#21894)) ;
#4673=EDGE_LOOP('',(#21895,#21896,#21897,#21898)) ;
#4674=EDGE_LOOP('',(#21899,#21900)) ;
#4675=EDGE_LOOP('',(#21901,#21902)) ;
#4676=EDGE_LOOP('',(#21903,#21904,#21905,#21906)) ;
#4677=EDGE_LOOP('',(#21907,#21908,#21909,#21910)) ;
#4678=EDGE_LOOP('',(#21911,#21912)) ;
#4679=EDGE_LOOP('',(#21913,#21914,#21915,#21916)) ;
#4680=EDGE_LOOP('',(#21917,#21918)) ;
#4681=EDGE_LOOP('',(#21919,#21920,#21921,#21922)) ;
#4682=EDGE_LOOP('',(#21923,#21924,#21925,#21926)) ;
#4683=EDGE_LOOP('',(#21927,#21928,#21929,#21930)) ;
#4684=EDGE_LOOP('',(#21931,#21932,#21933,#21934)) ;
#4685=EDGE_LOOP('',(#21935,#21936,#21937,#21938)) ;
#4686=EDGE_LOOP('',(#21939,#21940,#21941,#21942)) ;
#4687=EDGE_LOOP('',(#21943,#21944,#21945,#21946)) ;
#4688=EDGE_LOOP('',(#21947,#21948,#21949,#21950)) ;
#4689=EDGE_LOOP('',(#21951,#21952,#21953,#21954)) ;
#4690=EDGE_LOOP('',(#21955,#21956,#21957,#21958)) ;
#4691=EDGE_LOOP('',(#21959,#21960,#21961,#21962)) ;
#4692=EDGE_LOOP('',(#21963,#21964,#21965,#21966)) ;
#4693=EDGE_LOOP('',(#21967,#21968,#21969,#21970)) ;
#4694=EDGE_LOOP('',(#21971,#21972,#21973,#21974)) ;
#4695=EDGE_LOOP('',(#21975,#21976,#21977,#21978)) ;
#4696=EDGE_LOOP('',(#21979,#21980,#21981,#21982,#21983,#21984,#21985,#21986,
#21987,#21988,#21989,#21990)) ;
#4697=EDGE_LOOP('',(#21991,#21992,#21993,#21994)) ;
#4698=EDGE_LOOP('',(#21995,#21996,#21997,#21998)) ;
#4699=EDGE_LOOP('',(#21999,#22000,#22001,#22002,#22003,#22004,#22005,#22006,
#22007,#22008,#22009,#22010)) ;
#4700=EDGE_LOOP('',(#22011,#22012,#22013,#22014)) ;
#4701=EDGE_LOOP('',(#22015,#22016,#22017,#22018)) ;
#4702=EDGE_LOOP('',(#22019,#22020,#22021,#22022)) ;
#4703=EDGE_LOOP('',(#22023,#22024,#22025,#22026)) ;
#4704=EDGE_LOOP('',(#22027,#22028,#22029,#22030)) ;
#4705=EDGE_LOOP('',(#22031,#22032,#22033,#22034)) ;
#4706=EDGE_LOOP('',(#22035,#22036,#22037,#22038)) ;
#4707=EDGE_LOOP('',(#22039,#22040,#22041,#22042)) ;
#4708=EDGE_LOOP('',(#22043,#22044,#22045,#22046)) ;
#4709=EDGE_LOOP('',(#22047,#22048)) ;
#4710=EDGE_LOOP('',(#22049,#22050)) ;
#4711=EDGE_LOOP('',(#22051,#22052)) ;
#4712=EDGE_LOOP('',(#22053,#22054,#22055,#22056)) ;
#4713=EDGE_LOOP('',(#22057,#22058,#22059,#22060,#22061,#22062,#22063,#22064,
#22065,#22066,#22067,#22068)) ;
#4714=EDGE_LOOP('',(#22069,#22070)) ;
#4715=EDGE_LOOP('',(#22071,#22072,#22073,#22074)) ;
#4716=EDGE_LOOP('',(#22075,#22076,#22077,#22078)) ;
#4717=EDGE_LOOP('',(#22079,#22080,#22081,#22082)) ;
#4718=EDGE_LOOP('',(#22083,#22084,#22085,#22086)) ;
#6703=LINE('',#43764,#9175) ;
#6704=LINE('',#43770,#9176) ;
#6705=LINE('',#43776,#9177) ;
#6706=LINE('',#43782,#9178) ;
#6707=LINE('',#43788,#9179) ;
#6708=LINE('',#43794,#9180) ;
#6709=LINE('',#43799,#9181) ;
#6710=LINE('',#43803,#9182) ;
#6711=LINE('',#43808,#9183) ;
#6712=LINE('',#43810,#9184) ;
#6713=LINE('',#43812,#9185) ;
#6714=LINE('',#43813,#9186) ;
#6715=LINE('',#43815,#9187) ;
#6716=LINE('',#43817,#9188) ;
#6717=LINE('',#43819,#9189) ;
#6718=LINE('',#43820,#9190) ;
#6719=LINE('',#43823,#9191) ;
#6720=LINE('',#43825,#9192) ;
#6721=LINE('',#43826,#9193) ;
#6722=LINE('',#43828,#9194) ;
#6723=LINE('',#43830,#9195) ;
#6724=LINE('',#43832,#9196) ;
#6725=LINE('',#43838,#9197) ;
#6726=LINE('',#43844,#9198) ;
#6727=LINE('',#43849,#9199) ;
#6728=LINE('',#43853,#9200) ;
#6729=LINE('',#43858,#9201) ;
#6730=LINE('',#43860,#9202) ;
#6731=LINE('',#43862,#9203) ;
#6732=LINE('',#43863,#9204) ;
#6733=LINE('',#43865,#9205) ;
#6734=LINE('',#43867,#9206) ;
#6735=LINE('',#43869,#9207) ;
#6736=LINE('',#43870,#9208) ;
#6737=LINE('',#43873,#9209) ;
#6738=LINE('',#43875,#9210) ;
#6739=LINE('',#43876,#9211) ;
#6740=LINE('',#43878,#9212) ;
#6741=LINE('',#43880,#9213) ;
#6742=LINE('',#43882,#9214) ;
#6743=LINE('',#43888,#9215) ;
#6744=LINE('',#43894,#9216) ;
#6745=LINE('',#43900,#9217) ;
#6746=LINE('',#43906,#9218) ;
#6747=LINE('',#43912,#9219) ;
#6748=LINE('',#43914,#9220) ;
#6749=LINE('',#43916,#9221) ;
#6750=LINE('',#43918,#9222) ;
#6751=LINE('',#43919,#9223) ;
#6752=LINE('',#43926,#9224) ;
#6753=LINE('',#43931,#9225) ;
#6754=LINE('',#43937,#9226) ;
#6755=LINE('',#43939,#9227) ;
#6756=LINE('',#43941,#9228) ;
#6757=LINE('',#43942,#9229) ;
#6758=LINE('',#43945,#9230) ;
#6759=LINE('',#43947,#9231) ;
#6760=LINE('',#43948,#9232) ;
#6761=LINE('',#43951,#9233) ;
#6762=LINE('',#43953,#9234) ;
#6763=LINE('',#43954,#9235) ;
#6764=LINE('',#43956,#9236) ;
#6765=LINE('',#43957,#9237) ;
#6766=LINE('',#43961,#9238) ;
#6767=LINE('',#43963,#9239) ;
#6768=LINE('',#43965,#9240) ;
#6769=LINE('',#43966,#9241) ;
#6770=LINE('',#43969,#9242) ;
#6771=LINE('',#43971,#9243) ;
#6772=LINE('',#43972,#9244) ;
#6773=LINE('',#43975,#9245) ;
#6774=LINE('',#43977,#9246) ;
#6775=LINE('',#43978,#9247) ;
#6776=LINE('',#43981,#9248) ;
#6777=LINE('',#43983,#9249) ;
#6778=LINE('',#43985,#9250) ;
#6779=LINE('',#43986,#9251) ;
#6780=LINE('',#43991,#9252) ;
#6781=LINE('',#43993,#9253) ;
#6782=LINE('',#43995,#9254) ;
#6783=LINE('',#43996,#9255) ;
#6784=LINE('',#44003,#9256) ;
#6785=LINE('',#44005,#9257) ;
#6786=LINE('',#44007,#9258) ;
#6787=LINE('',#44008,#9259) ;
#6788=LINE('',#44013,#9260) ;
#6789=LINE('',#44015,#9261) ;
#6790=LINE('',#44017,#9262) ;
#6791=LINE('',#44018,#9263) ;
#6792=LINE('',#44020,#9264) ;
#6793=LINE('',#44022,#9265) ;
#6794=LINE('',#44023,#9266) ;
#6795=LINE('',#44027,#9267) ;
#6796=LINE('',#44029,#9268) ;
#6797=LINE('',#44030,#9269) ;
#6798=LINE('',#44032,#9270) ;
#6799=LINE('',#44034,#9271) ;
#6800=LINE('',#44036,#9272) ;
#6801=LINE('',#44037,#9273) ;
#6802=LINE('',#44039,#9274) ;
#6803=LINE('',#44042,#9275) ;
#6804=LINE('',#44046,#9276) ;
#6805=LINE('',#44047,#9277) ;
#6806=LINE('',#44050,#9278) ;
#6807=LINE('',#44052,#9279) ;
#6808=LINE('',#44056,#9280) ;
#6809=LINE('',#44058,#9281) ;
#6810=LINE('',#44059,#9282) ;
#6811=LINE('',#44063,#9283) ;
#6812=LINE('',#44065,#9284) ;
#6813=LINE('',#44067,#9285) ;
#6814=LINE('',#44068,#9286) ;
#6815=LINE('',#44072,#9287) ;
#6816=LINE('',#44074,#9288) ;
#6817=LINE('',#44076,#9289) ;
#6818=LINE('',#44077,#9290) ;
#6819=LINE('',#44081,#9291) ;
#6820=LINE('',#44083,#9292) ;
#6821=LINE('',#44085,#9293) ;
#6822=LINE('',#44086,#9294) ;
#6823=LINE('',#44089,#9295) ;
#6824=LINE('',#44091,#9296) ;
#6825=LINE('',#44092,#9297) ;
#6826=LINE('',#44096,#9298) ;
#6827=LINE('',#44098,#9299) ;
#6828=LINE('',#44100,#9300) ;
#6829=LINE('',#44104,#9301) ;
#6830=LINE('',#44106,#9302) ;
#6831=LINE('',#44107,#9303) ;
#6832=LINE('',#44112,#9304) ;
#6833=LINE('',#44114,#9305) ;
#6834=LINE('',#44116,#9306) ;
#6835=LINE('',#44118,#9307) ;
#6836=LINE('',#44120,#9308) ;
#6837=LINE('',#44121,#9309) ;
#6838=LINE('',#44123,#9310) ;
#6839=LINE('',#44124,#9311) ;
#6840=LINE('',#44126,#9312) ;
#6841=LINE('',#44128,#9313) ;
#6842=LINE('',#44130,#9314) ;
#6843=LINE('',#44132,#9315) ;
#6844=LINE('',#44134,#9316) ;
#6845=LINE('',#44136,#9317) ;
#6846=LINE('',#44137,#9318) ;
#6847=LINE('',#44140,#9319) ;
#6848=LINE('',#44142,#9320) ;
#6849=LINE('',#44143,#9321) ;
#6850=LINE('',#44145,#9322) ;
#6851=LINE('',#44147,#9323) ;
#6852=LINE('',#44148,#9324) ;
#6853=LINE('',#44149,#9325) ;
#6854=LINE('',#44154,#9326) ;
#6855=LINE('',#44155,#9327) ;
#6856=LINE('',#44158,#9328) ;
#6857=LINE('',#44159,#9329) ;
#6858=LINE('',#44162,#9330) ;
#6859=LINE('',#44163,#9331) ;
#6860=LINE('',#44166,#9332) ;
#6861=LINE('',#44168,#9333) ;
#6862=LINE('',#44169,#9334) ;
#6863=LINE('',#44172,#9335) ;
#6864=LINE('',#44173,#9336) ;
#6865=LINE('',#44176,#9337) ;
#6866=LINE('',#44178,#9338) ;
#6867=LINE('',#44179,#9339) ;
#6868=LINE('',#44182,#9340) ;
#6869=LINE('',#44183,#9341) ;
#6870=LINE('',#44185,#9342) ;
#6871=LINE('',#44187,#9343) ;
#6872=LINE('',#44188,#9344) ;
#6873=LINE('',#44191,#9345) ;
#6874=LINE('',#44192,#9346) ;
#6875=LINE('',#44201,#9347) ;
#6876=LINE('',#44202,#9348) ;
#6877=LINE('',#44204,#9349) ;
#6878=LINE('',#44205,#9350) ;
#6879=LINE('',#44208,#9351) ;
#6880=LINE('',#44210,#9352) ;
#6881=LINE('',#44211,#9353) ;
#6882=LINE('',#44213,#9354) ;
#6883=LINE('',#44214,#9355) ;
#6884=LINE('',#44216,#9356) ;
#6885=LINE('',#44219,#9357) ;
#6886=LINE('',#44222,#9358) ;
#6887=LINE('',#44235,#9359) ;
#6888=LINE('',#44237,#9360) ;
#6889=LINE('',#44239,#9361) ;
#6890=LINE('',#44241,#9362) ;
#6891=LINE('',#44244,#9363) ;
#6892=LINE('',#44246,#9364) ;
#6893=LINE('',#44247,#9365) ;
#6894=LINE('',#44251,#9366) ;
#6895=LINE('',#44253,#9367) ;
#6896=LINE('',#44255,#9368) ;
#6897=LINE('',#44256,#9369) ;
#6898=LINE('',#44260,#9370) ;
#6899=LINE('',#44262,#9371) ;
#6900=LINE('',#44264,#9372) ;
#6901=LINE('',#44265,#9373) ;
#6902=LINE('',#44267,#9374) ;
#6903=LINE('',#44268,#9375) ;
#6904=LINE('',#44272,#9376) ;
#6905=LINE('',#44273,#9377) ;
#6906=LINE('',#44274,#9378) ;
#6907=LINE('',#44276,#9379) ;
#6908=LINE('',#44277,#9380) ;
#6909=LINE('',#44279,#9381) ;
#6910=LINE('',#44281,#9382) ;
#6911=LINE('',#44285,#9383) ;
#6912=LINE('',#44287,#9384) ;
#6913=LINE('',#44289,#9385) ;
#6914=LINE('',#44290,#9386) ;
#6915=LINE('',#44292,#9387) ;
#6916=LINE('',#44293,#9388) ;
#6917=LINE('',#44295,#9389) ;
#6918=LINE('',#44297,#9390) ;
#6919=LINE('',#44301,#9391) ;
#6920=LINE('',#44303,#9392) ;
#6921=LINE('',#44305,#9393) ;
#6922=LINE('',#44306,#9394) ;
#6923=LINE('',#44308,#9395) ;
#6924=LINE('',#44309,#9396) ;
#6925=LINE('',#44311,#9397) ;
#6926=LINE('',#44313,#9398) ;
#6927=LINE('',#44325,#9399) ;
#6928=LINE('',#44328,#9400) ;
#6929=LINE('',#44338,#9401) ;
#6930=LINE('',#44340,#9402) ;
#6931=LINE('',#44344,#9403) ;
#6932=LINE('',#44349,#9404) ;
#6933=LINE('',#44351,#9405) ;
#6934=LINE('',#44353,#9406) ;
#6935=LINE('',#44356,#9407) ;
#6936=LINE('',#44358,#9408) ;
#6937=LINE('',#44359,#9409) ;
#6938=LINE('',#44361,#9410) ;
#6939=LINE('',#44362,#9411) ;
#6940=LINE('',#44366,#9412) ;
#6941=LINE('',#44368,#9413) ;
#6942=LINE('',#44371,#9414) ;
#6943=LINE('',#44372,#9415) ;
#6944=LINE('',#44375,#9416) ;
#6945=LINE('',#44377,#9417) ;
#6946=LINE('',#44378,#9418) ;
#6947=LINE('',#44382,#9419) ;
#6948=LINE('',#44384,#9420) ;
#6949=LINE('',#44386,#9421) ;
#6950=LINE('',#44387,#9422) ;
#6951=LINE('',#44391,#9423) ;
#6952=LINE('',#44393,#9424) ;
#6953=LINE('',#44395,#9425) ;
#6954=LINE('',#44396,#9426) ;
#6955=LINE('',#44398,#9427) ;
#6956=LINE('',#44399,#9428) ;
#6957=LINE('',#44400,#9429) ;
#6958=LINE('',#44402,#9430) ;
#6959=LINE('',#44404,#9431) ;
#6960=LINE('',#44406,#9432) ;
#6961=LINE('',#44413,#9433) ;
#6962=LINE('',#44416,#9434) ;
#6963=LINE('',#44419,#9435) ;
#6964=LINE('',#44421,#9436) ;
#6965=LINE('',#44422,#9437) ;
#6966=LINE('',#44425,#9438) ;
#6967=LINE('',#44426,#9439) ;
#6968=LINE('',#44429,#9440) ;
#6969=LINE('',#44430,#9441) ;
#6970=LINE('',#44432,#9442) ;
#6971=LINE('',#44437,#9443) ;
#6972=LINE('',#44439,#9444) ;
#6973=LINE('',#44441,#9445) ;
#6974=LINE('',#44442,#9446) ;
#6975=LINE('',#44447,#9447) ;
#6976=LINE('',#44448,#9448) ;
#6977=LINE('',#44451,#9449) ;
#6978=LINE('',#44452,#9450) ;
#6979=LINE('',#44456,#9451) ;
#6980=LINE('',#44458,#9452) ;
#6981=LINE('',#44464,#9453) ;
#6982=LINE('',#44469,#9454) ;
#6983=LINE('',#44471,#9455) ;
#6984=LINE('',#44472,#9456) ;
#6985=LINE('',#44477,#9457) ;
#6986=LINE('',#44479,#9458) ;
#6987=LINE('',#44481,#9459) ;
#6988=LINE('',#44482,#9460) ;
#6989=LINE('',#44485,#9461) ;
#6990=LINE('',#44487,#9462) ;
#6991=LINE('',#44488,#9463) ;
#6992=LINE('',#44497,#9464) ;
#6993=LINE('',#44500,#9465) ;
#6994=LINE('',#44503,#9466) ;
#6995=LINE('',#44505,#9467) ;
#6996=LINE('',#44506,#9468) ;
#6997=LINE('',#44509,#9469) ;
#6998=LINE('',#44512,#9470) ;
#6999=LINE('',#44517,#9471) ;
#7000=LINE('',#44519,#9472) ;
#7001=LINE('',#44521,#9473) ;
#7002=LINE('',#44522,#9474) ;
#7003=LINE('',#44525,#9475) ;
#7004=LINE('',#44527,#9476) ;
#7005=LINE('',#44528,#9477) ;
#7006=LINE('',#44537,#9478) ;
#7007=LINE('',#44539,#9479) ;
#7008=LINE('',#44544,#9480) ;
#7009=LINE('',#44547,#9481) ;
#7010=LINE('',#44549,#9482) ;
#7011=LINE('',#44550,#9483) ;
#7012=LINE('',#44552,#9484) ;
#7013=LINE('',#44557,#9485) ;
#7014=LINE('',#44559,#9486) ;
#7015=LINE('',#44561,#9487) ;
#7016=LINE('',#44562,#9488) ;
#7017=LINE('',#44567,#9489) ;
#7018=LINE('',#44570,#9490) ;
#7019=LINE('',#44572,#9491) ;
#7020=LINE('',#44577,#9492) ;
#7021=LINE('',#44579,#9493) ;
#7022=LINE('',#44584,#9494) ;
#7023=LINE('',#44587,#9495) ;
#7024=LINE('',#44589,#9496) ;
#7025=LINE('',#44590,#9497) ;
#7026=LINE('',#44592,#9498) ;
#7027=LINE('',#44597,#9499) ;
#7028=LINE('',#44599,#9500) ;
#7029=LINE('',#44601,#9501) ;
#7030=LINE('',#44602,#9502) ;
#7031=LINE('',#44611,#9503) ;
#7032=LINE('',#44615,#9504) ;
#7033=LINE('',#44618,#9505) ;
#7034=LINE('',#44620,#9506) ;
#7035=LINE('',#44625,#9507) ;
#7036=LINE('',#44627,#9508) ;
#7037=LINE('',#44629,#9509) ;
#7038=LINE('',#44630,#9510) ;
#7039=LINE('',#44639,#9511) ;
#7040=LINE('',#44643,#9512) ;
#7041=LINE('',#44646,#9513) ;
#7042=LINE('',#44648,#9514) ;
#7043=LINE('',#44653,#9515) ;
#7044=LINE('',#44655,#9516) ;
#7045=LINE('',#44657,#9517) ;
#7046=LINE('',#44658,#9518) ;
#7047=LINE('',#44667,#9519) ;
#7048=LINE('',#44669,#9520) ;
#7049=LINE('',#44671,#9521) ;
#7050=LINE('',#44672,#9522) ;
#7051=LINE('',#44675,#9523) ;
#7052=LINE('',#44677,#9524) ;
#7053=LINE('',#44678,#9525) ;
#7054=LINE('',#44681,#9526) ;
#7055=LINE('',#44683,#9527) ;
#7056=LINE('',#44684,#9528) ;
#7057=LINE('',#44686,#9529) ;
#7058=LINE('',#44687,#9530) ;
#7059=LINE('',#44693,#9531) ;
#7060=LINE('',#44695,#9532) ;
#7061=LINE('',#44697,#9533) ;
#7062=LINE('',#44698,#9534) ;
#7063=LINE('',#44702,#9535) ;
#7064=LINE('',#44704,#9536) ;
#7065=LINE('',#44706,#9537) ;
#7066=LINE('',#44707,#9538) ;
#7067=LINE('',#44709,#9539) ;
#7068=LINE('',#44710,#9540) ;
#7069=LINE('',#44712,#9541) ;
#7070=LINE('',#44714,#9542) ;
#7071=LINE('',#44719,#9543) ;
#7072=LINE('',#44721,#9544) ;
#7073=LINE('',#44723,#9545) ;
#7074=LINE('',#44724,#9546) ;
#7075=LINE('',#44727,#9547) ;
#7076=LINE('',#44729,#9548) ;
#7077=LINE('',#44730,#9549) ;
#7078=LINE('',#44733,#9550) ;
#7079=LINE('',#44735,#9551) ;
#7080=LINE('',#44736,#9552) ;
#7081=LINE('',#44739,#9553) ;
#7082=LINE('',#44741,#9554) ;
#7083=LINE('',#44743,#9555) ;
#7084=LINE('',#44745,#9556) ;
#7085=LINE('',#44747,#9557) ;
#7086=LINE('',#44749,#9558) ;
#7087=LINE('',#44751,#9559) ;
#7088=LINE('',#44753,#9560) ;
#7089=LINE('',#44754,#9561) ;
#7090=LINE('',#44757,#9562) ;
#7091=LINE('',#44758,#9563) ;
#7092=LINE('',#44761,#9564) ;
#7093=LINE('',#44762,#9565) ;
#7094=LINE('',#44765,#9566) ;
#7095=LINE('',#44767,#9567) ;
#7096=LINE('',#44769,#9568) ;
#7097=LINE('',#44771,#9569) ;
#7098=LINE('',#44773,#9570) ;
#7099=LINE('',#44775,#9571) ;
#7100=LINE('',#44776,#9572) ;
#7101=LINE('',#44778,#9573) ;
#7102=LINE('',#44779,#9574) ;
#7103=LINE('',#44782,#9575) ;
#7104=LINE('',#44784,#9576) ;
#7105=LINE('',#44786,#9577) ;
#7106=LINE('',#44788,#9578) ;
#7107=LINE('',#44793,#9579) ;
#7108=LINE('',#44797,#9580) ;
#7109=LINE('',#44800,#9581) ;
#7110=LINE('',#44801,#9582) ;
#7111=LINE('',#44808,#9583) ;
#7112=LINE('',#44811,#9584) ;
#7113=LINE('',#44813,#9585) ;
#7114=LINE('',#44814,#9586) ;
#7115=LINE('',#44819,#9587) ;
#7116=LINE('',#44823,#9588) ;
#7117=LINE('',#44827,#9589) ;
#7118=LINE('',#44831,#9590) ;
#7119=LINE('',#44834,#9591) ;
#7120=LINE('',#44836,#9592) ;
#7121=LINE('',#44838,#9593) ;
#7122=LINE('',#44840,#9594) ;
#9175=VECTOR('',#34776,0.65) ;
#9176=VECTOR('',#34783,0.65) ;
#9177=VECTOR('',#34790,0.65) ;
#9178=VECTOR('',#34797,0.65) ;
#9179=VECTOR('',#34804,0.65) ;
#9180=VECTOR('',#34811,0.65) ;
#9181=VECTOR('',#34816,1.) ;
#9182=VECTOR('',#34819,1.) ;
#9183=VECTOR('',#34824,1.) ;
#9184=VECTOR('',#34825,1.) ;
#9185=VECTOR('',#34826,1.) ;
#9186=VECTOR('',#34827,1.) ;
#9187=VECTOR('',#34830,1.) ;
#9188=VECTOR('',#34831,1.) ;
#9189=VECTOR('',#34832,1.) ;
#9190=VECTOR('',#34833,1.) ;
#9191=VECTOR('',#34836,1.) ;
#9192=VECTOR('',#34837,1.) ;
#9193=VECTOR('',#34838,1.) ;
#9194=VECTOR('',#34841,1.) ;
#9195=VECTOR('',#34844,1.) ;
#9196=VECTOR('',#34847,1.) ;
#9197=VECTOR('',#34854,0.65) ;
#9198=VECTOR('',#34861,0.65) ;
#9199=VECTOR('',#34866,1.) ;
#9200=VECTOR('',#34869,1.) ;
#9201=VECTOR('',#34874,1.) ;
#9202=VECTOR('',#34875,1.) ;
#9203=VECTOR('',#34876,1.) ;
#9204=VECTOR('',#34877,1.) ;
#9205=VECTOR('',#34880,1.) ;
#9206=VECTOR('',#34881,1.) ;
#9207=VECTOR('',#34882,1.) ;
#9208=VECTOR('',#34883,1.) ;
#9209=VECTOR('',#34886,1.) ;
#9210=VECTOR('',#34887,1.) ;
#9211=VECTOR('',#34888,1.) ;
#9212=VECTOR('',#34891,1.) ;
#9213=VECTOR('',#34894,1.) ;
#9214=VECTOR('',#34897,1.) ;
#9215=VECTOR('',#34904,1.28) ;
#9216=VECTOR('',#34911,1.28) ;
#9217=VECTOR('',#34918,1.2) ;
#9218=VECTOR('',#34925,1.5) ;
#9219=VECTOR('',#34932,1.) ;
#9220=VECTOR('',#34933,1.) ;
#9221=VECTOR('',#34934,1.) ;
#9222=VECTOR('',#34935,1.) ;
#9223=VECTOR('',#34936,1.) ;
#9224=VECTOR('',#34943,1.2) ;
#9225=VECTOR('',#34950,1.5) ;
#9226=VECTOR('',#34957,1.) ;
#9227=VECTOR('',#34958,1.) ;
#9228=VECTOR('',#34959,1.) ;
#9229=VECTOR('',#34960,1.) ;
#9230=VECTOR('',#34963,1.) ;
#9231=VECTOR('',#34964,1.) ;
#9232=VECTOR('',#34965,1.) ;
#9233=VECTOR('',#34968,1.) ;
#9234=VECTOR('',#34969,1.) ;
#9235=VECTOR('',#34970,1.) ;
#9236=VECTOR('',#34973,1.) ;
#9237=VECTOR('',#34974,1.) ;
#9238=VECTOR('',#34977,1.) ;
#9239=VECTOR('',#34978,1.) ;
#9240=VECTOR('',#34979,1.) ;
#9241=VECTOR('',#34980,1.) ;
#9242=VECTOR('',#34983,1.) ;
#9243=VECTOR('',#34984,1.) ;
#9244=VECTOR('',#34985,1.) ;
#9245=VECTOR('',#34988,1.) ;
#9246=VECTOR('',#34989,1.) ;
#9247=VECTOR('',#34990,1.) ;
#9248=VECTOR('',#34993,1.) ;
#9249=VECTOR('',#34994,1.) ;
#9250=VECTOR('',#34995,1.) ;
#9251=VECTOR('',#34996,1.) ;
#9252=VECTOR('',#35001,1.) ;
#9253=VECTOR('',#35002,1.) ;
#9254=VECTOR('',#35003,1.) ;
#9255=VECTOR('',#35004,1.) ;
#9256=VECTOR('',#35011,1.) ;
#9257=VECTOR('',#35012,1.) ;
#9258=VECTOR('',#35013,1.) ;
#9259=VECTOR('',#35014,1.) ;
#9260=VECTOR('',#35019,1.) ;
#9261=VECTOR('',#35020,1.) ;
#9262=VECTOR('',#35021,1.) ;
#9263=VECTOR('',#35022,1.) ;
#9264=VECTOR('',#35023,1.) ;
#9265=VECTOR('',#35024,1.) ;
#9266=VECTOR('',#35025,1.) ;
#9267=VECTOR('',#35028,1.) ;
#9268=VECTOR('',#35029,1.) ;
#9269=VECTOR('',#35030,1.) ;
#9270=VECTOR('',#35031,1.) ;
#9271=VECTOR('',#35032,1.) ;
#9272=VECTOR('',#35033,1.) ;
#9273=VECTOR('',#35034,1.) ;
#9274=VECTOR('',#35037,1.) ;
#9275=VECTOR('',#35040,1.) ;
#9276=VECTOR('',#35043,1.) ;
#9277=VECTOR('',#35044,1.) ;
#9278=VECTOR('',#35047,1.) ;
#9279=VECTOR('',#35048,1.) ;
#9280=VECTOR('',#35053,1.) ;
#9281=VECTOR('',#35054,1.) ;
#9282=VECTOR('',#35055,1.) ;
#9283=VECTOR('',#35058,1.) ;
#9284=VECTOR('',#35059,1.) ;
#9285=VECTOR('',#35060,1.) ;
#9286=VECTOR('',#35061,1.) ;
#9287=VECTOR('',#35064,1.) ;
#9288=VECTOR('',#35065,1.) ;
#9289=VECTOR('',#35066,1.) ;
#9290=VECTOR('',#35067,1.) ;
#9291=VECTOR('',#35070,1.) ;
#9292=VECTOR('',#35071,1.) ;
#9293=VECTOR('',#35072,1.) ;
#9294=VECTOR('',#35073,1.) ;
#9295=VECTOR('',#35076,1.) ;
#9296=VECTOR('',#35077,1.) ;
#9297=VECTOR('',#35078,1.) ;
#9298=VECTOR('',#35081,1.) ;
#9299=VECTOR('',#35082,1.) ;
#9300=VECTOR('',#35083,1.) ;
#9301=VECTOR('',#35088,1.) ;
#9302=VECTOR('',#35089,1.) ;
#9303=VECTOR('',#35090,1.) ;
#9304=VECTOR('',#35095,1.) ;
#9305=VECTOR('',#35096,1.) ;
#9306=VECTOR('',#35097,1.) ;
#9307=VECTOR('',#35098,1.) ;
#9308=VECTOR('',#35099,1.) ;
#9309=VECTOR('',#35100,1.) ;
#9310=VECTOR('',#35101,1.) ;
#9311=VECTOR('',#35102,1.) ;
#9312=VECTOR('',#35103,1.) ;
#9313=VECTOR('',#35104,1.) ;
#9314=VECTOR('',#35105,1.) ;
#9315=VECTOR('',#35106,1.) ;
#9316=VECTOR('',#35107,1.) ;
#9317=VECTOR('',#35108,1.) ;
#9318=VECTOR('',#35109,1.) ;
#9319=VECTOR('',#35110,1.) ;
#9320=VECTOR('',#35111,1.) ;
#9321=VECTOR('',#35112,1.) ;
#9322=VECTOR('',#35113,1.) ;
#9323=VECTOR('',#35114,1.) ;
#9324=VECTOR('',#35115,1.) ;
#9325=VECTOR('',#35116,1.) ;
#9326=VECTOR('',#35121,1.) ;
#9327=VECTOR('',#35122,1.) ;
#9328=VECTOR('',#35125,1.) ;
#9329=VECTOR('',#35126,1.) ;
#9330=VECTOR('',#35129,1.) ;
#9331=VECTOR('',#35130,1.) ;
#9332=VECTOR('',#35133,1.) ;
#9333=VECTOR('',#35134,1.) ;
#9334=VECTOR('',#35135,1.) ;
#9335=VECTOR('',#35138,1.) ;
#9336=VECTOR('',#35139,1.) ;
#9337=VECTOR('',#35142,1.) ;
#9338=VECTOR('',#35143,1.) ;
#9339=VECTOR('',#35144,1.) ;
#9340=VECTOR('',#35147,1.) ;
#9341=VECTOR('',#35148,1.) ;
#9342=VECTOR('',#35151,1.) ;
#9343=VECTOR('',#35152,1.) ;
#9344=VECTOR('',#35153,1.) ;
#9345=VECTOR('',#35156,1.) ;
#9346=VECTOR('',#35157,1.) ;
#9347=VECTOR('',#35168,1.) ;
#9348=VECTOR('',#35169,1.) ;
#9349=VECTOR('',#35170,1.) ;
#9350=VECTOR('',#35171,1.) ;
#9351=VECTOR('',#35174,1.) ;
#9352=VECTOR('',#35175,1.) ;
#9353=VECTOR('',#35176,1.) ;
#9354=VECTOR('',#35179,1.) ;
#9355=VECTOR('',#35180,1.) ;
#9356=VECTOR('',#35183,1.) ;
#9357=VECTOR('',#35188,1.) ;
#9358=VECTOR('',#35193,1.) ;
#9359=VECTOR('',#35210,3.) ;
#9360=VECTOR('',#35213,3.) ;
#9361=VECTOR('',#35216,2.6) ;
#9362=VECTOR('',#35219,2.6) ;
#9363=VECTOR('',#35222,1.) ;
#9364=VECTOR('',#35223,1.) ;
#9365=VECTOR('',#35224,1.) ;
#9366=VECTOR('',#35227,1.) ;
#9367=VECTOR('',#35228,1.) ;
#9368=VECTOR('',#35229,1.) ;
#9369=VECTOR('',#35230,1.) ;
#9370=VECTOR('',#35233,1.) ;
#9371=VECTOR('',#35234,1.) ;
#9372=VECTOR('',#35235,1.) ;
#9373=VECTOR('',#35236,1.) ;
#9374=VECTOR('',#35239,1.) ;
#9375=VECTOR('',#35240,1.) ;
#9376=VECTOR('',#35243,1.) ;
#9377=VECTOR('',#35244,1.) ;
#9378=VECTOR('',#35245,1.) ;
#9379=VECTOR('',#35248,1.) ;
#9380=VECTOR('',#35249,1.) ;
#9381=VECTOR('',#35252,1.) ;
#9382=VECTOR('',#35255,1.) ;
#9383=VECTOR('',#35258,1.) ;
#9384=VECTOR('',#35259,1.) ;
#9385=VECTOR('',#35260,1.) ;
#9386=VECTOR('',#35261,1.) ;
#9387=VECTOR('',#35264,1.) ;
#9388=VECTOR('',#35265,1.) ;
#9389=VECTOR('',#35268,1.) ;
#9390=VECTOR('',#35271,1.) ;
#9391=VECTOR('',#35274,1.) ;
#9392=VECTOR('',#35275,1.) ;
#9393=VECTOR('',#35276,1.) ;
#9394=VECTOR('',#35277,1.) ;
#9395=VECTOR('',#35280,1.) ;
#9396=VECTOR('',#35281,1.) ;
#9397=VECTOR('',#35284,1.) ;
#9398=VECTOR('',#35287,1.) ;
#9399=VECTOR('',#35302,1.5) ;
#9400=VECTOR('',#35307,1.2) ;
#9401=VECTOR('',#35320,1.5) ;
#9402=VECTOR('',#35323,1.2) ;
#9403=VECTOR('',#35326,1.) ;
#9404=VECTOR('',#35335,1.) ;
#9405=VECTOR('',#35338,1.) ;
#9406=VECTOR('',#35341,1.) ;
#9407=VECTOR('',#35344,1.) ;
#9408=VECTOR('',#35345,1.) ;
#9409=VECTOR('',#35346,1.) ;
#9410=VECTOR('',#35349,1.) ;
#9411=VECTOR('',#35350,1.) ;
#9412=VECTOR('',#35357,1.) ;
#9413=VECTOR('',#35360,1.) ;
#9414=VECTOR('',#35363,1.) ;
#9415=VECTOR('',#35364,1.) ;
#9416=VECTOR('',#35367,1.) ;
#9417=VECTOR('',#35368,1.) ;
#9418=VECTOR('',#35369,1.) ;
#9419=VECTOR('',#35372,1.) ;
#9420=VECTOR('',#35373,1.) ;
#9421=VECTOR('',#35374,1.) ;
#9422=VECTOR('',#35375,1.) ;
#9423=VECTOR('',#35378,1.) ;
#9424=VECTOR('',#35379,1.) ;
#9425=VECTOR('',#35380,1.) ;
#9426=VECTOR('',#35381,1.) ;
#9427=VECTOR('',#35384,1.) ;
#9428=VECTOR('',#35385,1.) ;
#9429=VECTOR('',#35386,1.) ;
#9430=VECTOR('',#35389,1.) ;
#9431=VECTOR('',#35392,1.) ;
#9432=VECTOR('',#35395,1.) ;
#9433=VECTOR('',#35402,1.) ;
#9434=VECTOR('',#35405,1.) ;
#9435=VECTOR('',#35408,1.) ;
#9436=VECTOR('',#35409,1.) ;
#9437=VECTOR('',#35410,1.) ;
#9438=VECTOR('',#35413,1.) ;
#9439=VECTOR('',#35414,1.) ;
#9440=VECTOR('',#35417,1.) ;
#9441=VECTOR('',#35418,1.) ;
#9442=VECTOR('',#35421,1.) ;
#9443=VECTOR('',#35426,1.) ;
#9444=VECTOR('',#35427,1.) ;
#9445=VECTOR('',#35428,1.) ;
#9446=VECTOR('',#35429,1.) ;
#9447=VECTOR('',#35434,1.) ;
#9448=VECTOR('',#35435,1.) ;
#9449=VECTOR('',#35438,1.) ;
#9450=VECTOR('',#35439,1.) ;
#9451=VECTOR('',#35444,1.) ;
#9452=VECTOR('',#35447,1.) ;
#9453=VECTOR('',#35454,1.) ;
#9454=VECTOR('',#35459,1.) ;
#9455=VECTOR('',#35462,1.) ;
#9456=VECTOR('',#35463,1.) ;
#9457=VECTOR('',#35468,1.) ;
#9458=VECTOR('',#35469,1.) ;
#9459=VECTOR('',#35470,1.) ;
#9460=VECTOR('',#35471,1.) ;
#9461=VECTOR('',#35474,1.) ;
#9462=VECTOR('',#35475,1.) ;
#9463=VECTOR('',#35476,1.) ;
#9464=VECTOR('',#35489,1.) ;
#9465=VECTOR('',#35492,1.) ;
#9466=VECTOR('',#35495,1.) ;
#9467=VECTOR('',#35496,1.) ;
#9468=VECTOR('',#35497,1.) ;
#9469=VECTOR('',#35500,1.) ;
#9470=VECTOR('',#35505,1.) ;
#9471=VECTOR('',#35510,1.) ;
#9472=VECTOR('',#35511,1.) ;
#9473=VECTOR('',#35512,1.) ;
#9474=VECTOR('',#35513,1.) ;
#9475=VECTOR('',#35516,1.) ;
#9476=VECTOR('',#35517,1.) ;
#9477=VECTOR('',#35518,1.) ;
#9478=VECTOR('',#35531,1.) ;
#9479=VECTOR('',#35532,1.) ;
#9480=VECTOR('',#35537,1.) ;
#9481=VECTOR('',#35540,1.) ;
#9482=VECTOR('',#35543,1.) ;
#9483=VECTOR('',#35544,1.) ;
#9484=VECTOR('',#35547,1.) ;
#9485=VECTOR('',#35552,1.) ;
#9486=VECTOR('',#35553,1.) ;
#9487=VECTOR('',#35554,1.) ;
#9488=VECTOR('',#35555,1.) ;
#9489=VECTOR('',#35560,1.) ;
#9490=VECTOR('',#35565,1.) ;
#9491=VECTOR('',#35568,1.) ;
#9492=VECTOR('',#35573,1.) ;
#9493=VECTOR('',#35574,1.) ;
#9494=VECTOR('',#35579,1.) ;
#9495=VECTOR('',#35582,1.) ;
#9496=VECTOR('',#35585,1.) ;
#9497=VECTOR('',#35586,1.) ;
#9498=VECTOR('',#35589,1.) ;
#9499=VECTOR('',#35594,1.) ;
#9500=VECTOR('',#35595,1.) ;
#9501=VECTOR('',#35596,1.) ;
#9502=VECTOR('',#35597,1.) ;
#9503=VECTOR('',#35610,1.) ;
#9504=VECTOR('',#35613,1.) ;
#9505=VECTOR('',#35618,1.) ;
#9506=VECTOR('',#35621,1.) ;
#9507=VECTOR('',#35626,1.) ;
#9508=VECTOR('',#35627,1.) ;
#9509=VECTOR('',#35628,1.) ;
#9510=VECTOR('',#35629,1.) ;
#9511=VECTOR('',#35642,1.) ;
#9512=VECTOR('',#35645,1.) ;
#9513=VECTOR('',#35650,1.) ;
#9514=VECTOR('',#35653,1.) ;
#9515=VECTOR('',#35658,1.) ;
#9516=VECTOR('',#35659,1.) ;
#9517=VECTOR('',#35660,1.) ;
#9518=VECTOR('',#35661,1.) ;
#9519=VECTOR('',#35674,1.) ;
#9520=VECTOR('',#35675,1.) ;
#9521=VECTOR('',#35676,1.) ;
#9522=VECTOR('',#35677,1.) ;
#9523=VECTOR('',#35680,1.) ;
#9524=VECTOR('',#35681,1.) ;
#9525=VECTOR('',#35682,1.) ;
#9526=VECTOR('',#35685,1.) ;
#9527=VECTOR('',#35686,1.) ;
#9528=VECTOR('',#35687,1.) ;
#9529=VECTOR('',#35690,1.) ;
#9530=VECTOR('',#35691,1.) ;
#9531=VECTOR('',#35698,1.) ;
#9532=VECTOR('',#35699,1.) ;
#9533=VECTOR('',#35700,1.) ;
#9534=VECTOR('',#35701,1.) ;
#9535=VECTOR('',#35704,1.) ;
#9536=VECTOR('',#35705,1.) ;
#9537=VECTOR('',#35706,1.) ;
#9538=VECTOR('',#35707,1.) ;
#9539=VECTOR('',#35710,1.) ;
#9540=VECTOR('',#35711,1.) ;
#9541=VECTOR('',#35714,1.) ;
#9542=VECTOR('',#35717,1.) ;
#9543=VECTOR('',#35722,1.) ;
#9544=VECTOR('',#35723,1.) ;
#9545=VECTOR('',#35724,1.) ;
#9546=VECTOR('',#35725,1.) ;
#9547=VECTOR('',#35728,1.) ;
#9548=VECTOR('',#35729,1.) ;
#9549=VECTOR('',#35730,1.) ;
#9550=VECTOR('',#35733,1.) ;
#9551=VECTOR('',#35734,1.) ;
#9552=VECTOR('',#35735,1.) ;
#9553=VECTOR('',#35738,1.) ;
#9554=VECTOR('',#35739,1.) ;
#9555=VECTOR('',#35740,1.) ;
#9556=VECTOR('',#35741,1.) ;
#9557=VECTOR('',#35742,1.) ;
#9558=VECTOR('',#35743,1.) ;
#9559=VECTOR('',#35744,1.) ;
#9560=VECTOR('',#35745,1.) ;
#9561=VECTOR('',#35746,1.) ;
#9562=VECTOR('',#35749,1.) ;
#9563=VECTOR('',#35750,1.) ;
#9564=VECTOR('',#35753,1.) ;
#9565=VECTOR('',#35754,1.) ;
#9566=VECTOR('',#35757,1.) ;
#9567=VECTOR('',#35758,1.) ;
#9568=VECTOR('',#35759,1.) ;
#9569=VECTOR('',#35760,1.) ;
#9570=VECTOR('',#35761,1.) ;
#9571=VECTOR('',#35762,1.) ;
#9572=VECTOR('',#35763,1.) ;
#9573=VECTOR('',#35766,1.) ;
#9574=VECTOR('',#35767,1.) ;
#9575=VECTOR('',#35772,1.) ;
#9576=VECTOR('',#35775,1.) ;
#9577=VECTOR('',#35778,1.) ;
#9578=VECTOR('',#35781,1.) ;
#9579=VECTOR('',#35786,1.) ;
#9580=VECTOR('',#35789,1.) ;
#9581=VECTOR('',#35794,1.) ;
#9582=VECTOR('',#35795,1.) ;
#9583=VECTOR('',#35804,1.) ;
#9584=VECTOR('',#35807,1.) ;
#9585=VECTOR('',#35808,1.) ;
#9586=VECTOR('',#35809,1.) ;
#9587=VECTOR('',#35814,1.) ;
#9588=VECTOR('',#35817,1.) ;
#9589=VECTOR('',#35820,1.) ;
#9590=VECTOR('',#35823,1.) ;
#9591=VECTOR('',#35828,1.) ;
#9592=VECTOR('',#35831,1.) ;
#9593=VECTOR('',#35834,1.) ;
#9594=VECTOR('',#35837,1.) ;
#10906=CIRCLE('',#29923,0.65) ;
#10907=CIRCLE('',#29924,0.65) ;
#10908=CIRCLE('',#29926,0.65) ;
#10909=CIRCLE('',#29927,0.65) ;
#10910=CIRCLE('',#29929,0.65) ;
#10911=CIRCLE('',#29930,0.65) ;
#10912=CIRCLE('',#29932,0.65) ;
#10913=CIRCLE('',#29933,0.65) ;
#10914=CIRCLE('',#29935,0.65) ;
#10915=CIRCLE('',#29936,0.65) ;
#10916=CIRCLE('',#29938,0.65) ;
#10917=CIRCLE('',#29939,0.65) ;
#10918=CIRCLE('',#29941,3.) ;
#10919=CIRCLE('',#29942,3.) ;
#10920=CIRCLE('',#29951,0.65) ;
#10921=CIRCLE('',#29952,0.65) ;
#10922=CIRCLE('',#29954,0.65) ;
#10923=CIRCLE('',#29955,0.65) ;
#10924=CIRCLE('',#29957,3.) ;
#10925=CIRCLE('',#29958,3.) ;
#10926=CIRCLE('',#29967,1.28) ;
#10927=CIRCLE('',#29968,1.28) ;
#10928=CIRCLE('',#29970,1.28) ;
#10929=CIRCLE('',#29971,1.28) ;
#10930=CIRCLE('',#29973,1.2) ;
#10931=CIRCLE('',#29974,1.2) ;
#10932=CIRCLE('',#29976,1.5) ;
#10933=CIRCLE('',#29977,1.5) ;
#10934=CIRCLE('',#29980,1.5) ;
#10935=CIRCLE('',#29982,1.2) ;
#10936=CIRCLE('',#29983,1.2) ;
#10937=CIRCLE('',#29985,1.5) ;
#10938=CIRCLE('',#29999,1.2) ;
#10939=CIRCLE('',#30002,3.) ;
#10940=CIRCLE('',#30006,3.) ;
#10941=CIRCLE('',#30008,3.) ;
#10942=CIRCLE('',#30015,3.) ;
#10943=CIRCLE('',#30017,3.) ;
#10944=CIRCLE('',#30020,3.) ;
#10945=CIRCLE('',#30030,2.6) ;
#10946=CIRCLE('',#30032,2.6) ;
#10947=CIRCLE('',#30037,3.) ;
#10948=CIRCLE('',#30043,3.) ;
#10949=CIRCLE('',#30044,2.6) ;
#10950=CIRCLE('',#30046,3.) ;
#10951=CIRCLE('',#30047,2.6) ;
#10952=CIRCLE('',#30070,1.2) ;
#10953=CIRCLE('',#30072,1.5) ;
#10954=CIRCLE('',#30073,1.2) ;
#10955=CIRCLE('',#30075,1.5) ;
#10956=CIRCLE('',#30078,1.5) ;
#10957=CIRCLE('',#30080,1.5) ;
#10958=CIRCLE('',#30081,1.2) ;
#10959=CIRCLE('',#30085,3.) ;
#10960=CIRCLE('',#30086,3.) ;
#10961=CIRCLE('',#30087,3.) ;
#10962=CIRCLE('',#30107,3.) ;
#10963=CIRCLE('',#30108,3.) ;
#10964=CIRCLE('',#30116,3.) ;
#10965=CIRCLE('',#30119,3.) ;
#10966=CIRCLE('',#30123,2.6) ;
#10967=CIRCLE('',#30125,2.6) ;
#10968=CIRCLE('',#30131,3.) ;
#10969=CIRCLE('',#30133,3.) ;
#10970=CIRCLE('',#30136,3.) ;
#10971=CIRCLE('',#30139,3.) ;
#10972=CIRCLE('',#30145,3.) ;
#10973=CIRCLE('',#30147,3.) ;
#10974=CIRCLE('',#30150,3.) ;
#10975=CIRCLE('',#30152,3.) ;
#10976=CIRCLE('',#30158,3.) ;
#10977=CIRCLE('',#30159,3.) ;
#10978=CIRCLE('',#30164,3.) ;
#10979=CIRCLE('',#30166,3.) ;
#10980=CIRCLE('',#30172,2.6) ;
#10981=CIRCLE('',#30174,2.6) ;
#10982=CIRCLE('',#30177,2.6) ;
#10983=CIRCLE('',#30178,2.6) ;
#10984=CIRCLE('',#30184,2.6) ;
#10985=CIRCLE('',#30186,2.6) ;
#10986=CIRCLE('',#30189,2.6) ;
#10987=CIRCLE('',#30190,2.6) ;
#10988=CIRCLE('',#30196,2.6) ;
#10989=CIRCLE('',#30198,2.6) ;
#10990=CIRCLE('',#30227,2.6) ;
#10991=CIRCLE('',#30228,2.6) ;
#10992=CIRCLE('',#30233,2.6) ;
#10993=CIRCLE('',#30236,2.6) ;
#10994=CIRCLE('',#30237,2.6) ;
#10995=CIRCLE('',#30238,2.6) ;
#10996=CIRCLE('',#30239,2.6) ;
#10997=CIRCLE('',#30240,2.6) ;
#12674=VERTEX_POINT('',#43761) ;
#12675=VERTEX_POINT('',#43763) ;
#12676=VERTEX_POINT('',#43767) ;
#12677=VERTEX_POINT('',#43769) ;
#12678=VERTEX_POINT('',#43773) ;
#12679=VERTEX_POINT('',#43775) ;
#12680=VERTEX_POINT('',#43779) ;
#12681=VERTEX_POINT('',#43781) ;
#12682=VERTEX_POINT('',#43785) ;
#12683=VERTEX_POINT('',#43787) ;
#12684=VERTEX_POINT('',#43791) ;
#12685=VERTEX_POINT('',#43793) ;
#12686=VERTEX_POINT('',#43797) ;
#12687=VERTEX_POINT('',#43798) ;
#12688=VERTEX_POINT('',#43800) ;
#12689=VERTEX_POINT('',#43802) ;
#12690=VERTEX_POINT('',#43806) ;
#12691=VERTEX_POINT('',#43807) ;
#12692=VERTEX_POINT('',#43809) ;
#12693=VERTEX_POINT('',#43811) ;
#12694=VERTEX_POINT('',#43816) ;
#12695=VERTEX_POINT('',#43818) ;
#12696=VERTEX_POINT('',#43822) ;
#12697=VERTEX_POINT('',#43824) ;
#12698=VERTEX_POINT('',#43835) ;
#12699=VERTEX_POINT('',#43837) ;
#12700=VERTEX_POINT('',#43841) ;
#12701=VERTEX_POINT('',#43843) ;
#12702=VERTEX_POINT('',#43847) ;
#12703=VERTEX_POINT('',#43848) ;
#12704=VERTEX_POINT('',#43850) ;
#12705=VERTEX_POINT('',#43852) ;
#12706=VERTEX_POINT('',#43856) ;
#12707=VERTEX_POINT('',#43857) ;
#12708=VERTEX_POINT('',#43859) ;
#12709=VERTEX_POINT('',#43861) ;
#12710=VERTEX_POINT('',#43866) ;
#12711=VERTEX_POINT('',#43868) ;
#12712=VERTEX_POINT('',#43872) ;
#12713=VERTEX_POINT('',#43874) ;
#12714=VERTEX_POINT('',#43885) ;
#12715=VERTEX_POINT('',#43887) ;
#12716=VERTEX_POINT('',#43891) ;
#12717=VERTEX_POINT('',#43893) ;
#12718=VERTEX_POINT('',#43897) ;
#12719=VERTEX_POINT('',#43899) ;
#12720=VERTEX_POINT('',#43903) ;
#12721=VERTEX_POINT('',#43905) ;
#12722=VERTEX_POINT('',#43910) ;
#12723=VERTEX_POINT('',#43911) ;
#12724=VERTEX_POINT('',#43913) ;
#12725=VERTEX_POINT('',#43915) ;
#12726=VERTEX_POINT('',#43917) ;
#12727=VERTEX_POINT('',#43920) ;
#12728=VERTEX_POINT('',#43923) ;
#12729=VERTEX_POINT('',#43925) ;
#12730=VERTEX_POINT('',#43929) ;
#12731=VERTEX_POINT('',#43935) ;
#12732=VERTEX_POINT('',#43936) ;
#12733=VERTEX_POINT('',#43938) ;
#12734=VERTEX_POINT('',#43940) ;
#12735=VERTEX_POINT('',#43944) ;
#12736=VERTEX_POINT('',#43946) ;
#12737=VERTEX_POINT('',#43950) ;
#12738=VERTEX_POINT('',#43952) ;
#12739=VERTEX_POINT('',#43959) ;
#12740=VERTEX_POINT('',#43960) ;
#12741=VERTEX_POINT('',#43962) ;
#12742=VERTEX_POINT('',#43964) ;
#12743=VERTEX_POINT('',#43968) ;
#12744=VERTEX_POINT('',#43970) ;
#12745=VERTEX_POINT('',#43974) ;
#12746=VERTEX_POINT('',#43976) ;
#12747=VERTEX_POINT('',#43980) ;
#12748=VERTEX_POINT('',#43982) ;
#12749=VERTEX_POINT('',#43984) ;
#12750=VERTEX_POINT('',#43989) ;
#12751=VERTEX_POINT('',#43990) ;
#12752=VERTEX_POINT('',#43992) ;
#12753=VERTEX_POINT('',#43994) ;
#12754=VERTEX_POINT('',#43998) ;
#12755=VERTEX_POINT('',#44001) ;
#12756=VERTEX_POINT('',#44002) ;
#12757=VERTEX_POINT('',#44004) ;
#12758=VERTEX_POINT('',#44006) ;
#12759=VERTEX_POINT('',#44010) ;
#12760=VERTEX_POINT('',#44012) ;
#12761=VERTEX_POINT('',#44014) ;
#12762=VERTEX_POINT('',#44016) ;
#12763=VERTEX_POINT('',#44019) ;
#12764=VERTEX_POINT('',#44021) ;
#12765=VERTEX_POINT('',#44025) ;
#12766=VERTEX_POINT('',#44026) ;
#12767=VERTEX_POINT('',#44028) ;
#12768=VERTEX_POINT('',#44031) ;
#12769=VERTEX_POINT('',#44033) ;
#12770=VERTEX_POINT('',#44035) ;
#12771=VERTEX_POINT('',#44041) ;
#12772=VERTEX_POINT('',#44043) ;
#12773=VERTEX_POINT('',#44045) ;
#12774=VERTEX_POINT('',#44049) ;
#12775=VERTEX_POINT('',#44051) ;
#12776=VERTEX_POINT('',#44055) ;
#12777=VERTEX_POINT('',#44057) ;
#12778=VERTEX_POINT('',#44061) ;
#12779=VERTEX_POINT('',#44062) ;
#12780=VERTEX_POINT('',#44064) ;
#12781=VERTEX_POINT('',#44066) ;
#12782=VERTEX_POINT('',#44070) ;
#12783=VERTEX_POINT('',#44071) ;
#12784=VERTEX_POINT('',#44073) ;
#12785=VERTEX_POINT('',#44075) ;
#12786=VERTEX_POINT('',#44079) ;
#12787=VERTEX_POINT('',#44080) ;
#12788=VERTEX_POINT('',#44082) ;
#12789=VERTEX_POINT('',#44084) ;
#12790=VERTEX_POINT('',#44088) ;
#12791=VERTEX_POINT('',#44090) ;
#12792=VERTEX_POINT('',#44094) ;
#12793=VERTEX_POINT('',#44095) ;
#12794=VERTEX_POINT('',#44097) ;
#12795=VERTEX_POINT('',#44099) ;
#12796=VERTEX_POINT('',#44103) ;
#12797=VERTEX_POINT('',#44105) ;
#12798=VERTEX_POINT('',#44110) ;
#12799=VERTEX_POINT('',#44111) ;
#12800=VERTEX_POINT('',#44113) ;
#12801=VERTEX_POINT('',#44115) ;
#12802=VERTEX_POINT('',#44117) ;
#12803=VERTEX_POINT('',#44119) ;
#12804=VERTEX_POINT('',#44122) ;
#12805=VERTEX_POINT('',#44125) ;
#12806=VERTEX_POINT('',#44127) ;
#12807=VERTEX_POINT('',#44129) ;
#12808=VERTEX_POINT('',#44131) ;
#12809=VERTEX_POINT('',#44133) ;
#12810=VERTEX_POINT('',#44135) ;
#12811=VERTEX_POINT('',#44138) ;
#12812=VERTEX_POINT('',#44139) ;
#12813=VERTEX_POINT('',#44141) ;
#12814=VERTEX_POINT('',#44144) ;
#12815=VERTEX_POINT('',#44146) ;
#12816=VERTEX_POINT('',#44151) ;
#12817=VERTEX_POINT('',#44153) ;
#12818=VERTEX_POINT('',#44157) ;
#12819=VERTEX_POINT('',#44161) ;
#12820=VERTEX_POINT('',#44165) ;
#12821=VERTEX_POINT('',#44167) ;
#12822=VERTEX_POINT('',#44171) ;
#12823=VERTEX_POINT('',#44175) ;
#12824=VERTEX_POINT('',#44177) ;
#12825=VERTEX_POINT('',#44181) ;
#12826=VERTEX_POINT('',#44186) ;
#12827=VERTEX_POINT('',#44190) ;
#12828=VERTEX_POINT('',#44194) ;
#12829=VERTEX_POINT('',#44197) ;
#12830=VERTEX_POINT('',#44200) ;
#12831=VERTEX_POINT('',#44203) ;
#12832=VERTEX_POINT('',#44207) ;
#12833=VERTEX_POINT('',#44209) ;
#12834=VERTEX_POINT('',#44225) ;
#12835=VERTEX_POINT('',#44227) ;
#12836=VERTEX_POINT('',#44230) ;
#12837=VERTEX_POINT('',#44232) ;
#12838=VERTEX_POINT('',#44243) ;
#12839=VERTEX_POINT('',#44245) ;
#12840=VERTEX_POINT('',#44249) ;
#12841=VERTEX_POINT('',#44250) ;
#12842=VERTEX_POINT('',#44252) ;
#12843=VERTEX_POINT('',#44254) ;
#12844=VERTEX_POINT('',#44258) ;
#12845=VERTEX_POINT('',#44259) ;
#12846=VERTEX_POINT('',#44261) ;
#12847=VERTEX_POINT('',#44263) ;
#12848=VERTEX_POINT('',#44270) ;
#12849=VERTEX_POINT('',#44271) ;
#12850=VERTEX_POINT('',#44283) ;
#12851=VERTEX_POINT('',#44284) ;
#12852=VERTEX_POINT('',#44286) ;
#12853=VERTEX_POINT('',#44288) ;
#12854=VERTEX_POINT('',#44299) ;
#12855=VERTEX_POINT('',#44300) ;
#12856=VERTEX_POINT('',#44302) ;
#12857=VERTEX_POINT('',#44304) ;
#12858=VERTEX_POINT('',#44316) ;
#12859=VERTEX_POINT('',#44319) ;
#12860=VERTEX_POINT('',#44321) ;
#12861=VERTEX_POINT('',#44324) ;
#12862=VERTEX_POINT('',#44330) ;
#12863=VERTEX_POINT('',#44333) ;
#12864=VERTEX_POINT('',#44335) ;
#12865=VERTEX_POINT('',#44342) ;
#12866=VERTEX_POINT('',#44343) ;
#12867=VERTEX_POINT('',#44355) ;
#12868=VERTEX_POINT('',#44357) ;
#12869=VERTEX_POINT('',#44370) ;
#12870=VERTEX_POINT('',#44374) ;
#12871=VERTEX_POINT('',#44376) ;
#12872=VERTEX_POINT('',#44380) ;
#12873=VERTEX_POINT('',#44381) ;
#12874=VERTEX_POINT('',#44383) ;
#12875=VERTEX_POINT('',#44385) ;
#12876=VERTEX_POINT('',#44389) ;
#12877=VERTEX_POINT('',#44390) ;
#12878=VERTEX_POINT('',#44392) ;
#12879=VERTEX_POINT('',#44394) ;
#12880=VERTEX_POINT('',#44409) ;
#12881=VERTEX_POINT('',#44410) ;
#12882=VERTEX_POINT('',#44412) ;
#12883=VERTEX_POINT('',#44414) ;
#12884=VERTEX_POINT('',#44418) ;
#12885=VERTEX_POINT('',#44420) ;
#12886=VERTEX_POINT('',#44424) ;
#12887=VERTEX_POINT('',#44428) ;
#12888=VERTEX_POINT('',#44435) ;
#12889=VERTEX_POINT('',#44436) ;
#12890=VERTEX_POINT('',#44438) ;
#12891=VERTEX_POINT('',#44440) ;
#12892=VERTEX_POINT('',#44444) ;
#12893=VERTEX_POINT('',#44445) ;
#12894=VERTEX_POINT('',#44450) ;
#12895=VERTEX_POINT('',#44454) ;
#12896=VERTEX_POINT('',#44461) ;
#12897=VERTEX_POINT('',#44462) ;
#12898=VERTEX_POINT('',#44466) ;
#12899=VERTEX_POINT('',#44467) ;
#12900=VERTEX_POINT('',#44475) ;
#12901=VERTEX_POINT('',#44476) ;
#12902=VERTEX_POINT('',#44478) ;
#12903=VERTEX_POINT('',#44480) ;
#12904=VERTEX_POINT('',#44484) ;
#12905=VERTEX_POINT('',#44486) ;
#12906=VERTEX_POINT('',#44495) ;
#12907=VERTEX_POINT('',#44496) ;
#12908=VERTEX_POINT('',#44498) ;
#12909=VERTEX_POINT('',#44502) ;
#12910=VERTEX_POINT('',#44504) ;
#12911=VERTEX_POINT('',#44508) ;
#12912=VERTEX_POINT('',#44515) ;
#12913=VERTEX_POINT('',#44516) ;
#12914=VERTEX_POINT('',#44518) ;
#12915=VERTEX_POINT('',#44520) ;
#12916=VERTEX_POINT('',#44524) ;
#12917=VERTEX_POINT('',#44526) ;
#12918=VERTEX_POINT('',#44535) ;
#12919=VERTEX_POINT('',#44536) ;
#12920=VERTEX_POINT('',#44538) ;
#12921=VERTEX_POINT('',#44542) ;
#12922=VERTEX_POINT('',#44543) ;
#12923=VERTEX_POINT('',#44545) ;
#12924=VERTEX_POINT('',#44555) ;
#12925=VERTEX_POINT('',#44556) ;
#12926=VERTEX_POINT('',#44558) ;
#12927=VERTEX_POINT('',#44560) ;
#12928=VERTEX_POINT('',#44564) ;
#12929=VERTEX_POINT('',#44566) ;
#12930=VERTEX_POINT('',#44575) ;
#12931=VERTEX_POINT('',#44576) ;
#12932=VERTEX_POINT('',#44578) ;
#12933=VERTEX_POINT('',#44582) ;
#12934=VERTEX_POINT('',#44583) ;
#12935=VERTEX_POINT('',#44585) ;
#12936=VERTEX_POINT('',#44595) ;
#12937=VERTEX_POINT('',#44596) ;
#12938=VERTEX_POINT('',#44598) ;
#12939=VERTEX_POINT('',#44600) ;
#12940=VERTEX_POINT('',#44609) ;
#12941=VERTEX_POINT('',#44610) ;
#12942=VERTEX_POINT('',#44612) ;
#12943=VERTEX_POINT('',#44614) ;
#12944=VERTEX_POINT('',#44623) ;
#12945=VERTEX_POINT('',#44624) ;
#12946=VERTEX_POINT('',#44626) ;
#12947=VERTEX_POINT('',#44628) ;
#12948=VERTEX_POINT('',#44637) ;
#12949=VERTEX_POINT('',#44638) ;
#12950=VERTEX_POINT('',#44640) ;
#12951=VERTEX_POINT('',#44642) ;
#12952=VERTEX_POINT('',#44651) ;
#12953=VERTEX_POINT('',#44652) ;
#12954=VERTEX_POINT('',#44654) ;
#12955=VERTEX_POINT('',#44656) ;
#12956=VERTEX_POINT('',#44665) ;
#12957=VERTEX_POINT('',#44666) ;
#12958=VERTEX_POINT('',#44668) ;
#12959=VERTEX_POINT('',#44670) ;
#12960=VERTEX_POINT('',#44674) ;
#12961=VERTEX_POINT('',#44676) ;
#12962=VERTEX_POINT('',#44680) ;
#12963=VERTEX_POINT('',#44682) ;
#12964=VERTEX_POINT('',#44691) ;
#12965=VERTEX_POINT('',#44692) ;
#12966=VERTEX_POINT('',#44694) ;
#12967=VERTEX_POINT('',#44696) ;
#12968=VERTEX_POINT('',#44700) ;
#12969=VERTEX_POINT('',#44701) ;
#12970=VERTEX_POINT('',#44703) ;
#12971=VERTEX_POINT('',#44705) ;
#12972=VERTEX_POINT('',#44717) ;
#12973=VERTEX_POINT('',#44718) ;
#12974=VERTEX_POINT('',#44720) ;
#12975=VERTEX_POINT('',#44722) ;
#12976=VERTEX_POINT('',#44726) ;
#12977=VERTEX_POINT('',#44728) ;
#12978=VERTEX_POINT('',#44732) ;
#12979=VERTEX_POINT('',#44734) ;
#12980=VERTEX_POINT('',#44738) ;
#12981=VERTEX_POINT('',#44740) ;
#12982=VERTEX_POINT('',#44742) ;
#12983=VERTEX_POINT('',#44744) ;
#12984=VERTEX_POINT('',#44746) ;
#12985=VERTEX_POINT('',#44748) ;
#12986=VERTEX_POINT('',#44750) ;
#12987=VERTEX_POINT('',#44752) ;
#12988=VERTEX_POINT('',#44756) ;
#12989=VERTEX_POINT('',#44760) ;
#12990=VERTEX_POINT('',#44764) ;
#12991=VERTEX_POINT('',#44766) ;
#12992=VERTEX_POINT('',#44768) ;
#12993=VERTEX_POINT('',#44770) ;
#12994=VERTEX_POINT('',#44772) ;
#12995=VERTEX_POINT('',#44774) ;
#12996=VERTEX_POINT('',#44791) ;
#12997=VERTEX_POINT('',#44792) ;
#12998=VERTEX_POINT('',#44794) ;
#12999=VERTEX_POINT('',#44796) ;
#13000=VERTEX_POINT('',#44805) ;
#13001=VERTEX_POINT('',#44806) ;
#13002=VERTEX_POINT('',#44810) ;
#13003=VERTEX_POINT('',#44812) ;
#13004=VERTEX_POINT('',#44816) ;
#13005=VERTEX_POINT('',#44818) ;
#13006=VERTEX_POINT('',#44820) ;
#13007=VERTEX_POINT('',#44822) ;
#13008=VERTEX_POINT('',#44824) ;
#13009=VERTEX_POINT('',#44826) ;
#13010=VERTEX_POINT('',#44828) ;
#13011=VERTEX_POINT('',#44830) ;
#15797=EDGE_CURVE('',#12674,#12674,#10906,.T.) ;
#15798=EDGE_CURVE('',#12674,#12675,#6703,.T.) ;
#15799=EDGE_CURVE('',#12675,#12675,#10907,.T.) ;
#15800=EDGE_CURVE('',#12676,#12676,#10908,.T.) ;
#15801=EDGE_CURVE('',#12676,#12677,#6704,.T.) ;
#15802=EDGE_CURVE('',#12677,#12677,#10909,.T.) ;
#15803=EDGE_CURVE('',#12678,#12678,#10910,.T.) ;
#15804=EDGE_CURVE('',#12678,#12679,#6705,.T.) ;
#15805=EDGE_CURVE('',#12679,#12679,#10911,.T.) ;
#15806=EDGE_CURVE('',#12680,#12680,#10912,.T.) ;
#15807=EDGE_CURVE('',#12680,#12681,#6706,.T.) ;
#15808=EDGE_CURVE('',#12681,#12681,#10913,.T.) ;
#15809=EDGE_CURVE('',#12682,#12682,#10914,.T.) ;
#15810=EDGE_CURVE('',#12682,#12683,#6707,.T.) ;
#15811=EDGE_CURVE('',#12683,#12683,#10915,.T.) ;
#15812=EDGE_CURVE('',#12684,#12684,#10916,.T.) ;
#15813=EDGE_CURVE('',#12684,#12685,#6708,.T.) ;
#15814=EDGE_CURVE('',#12685,#12685,#10917,.T.) ;
#15815=EDGE_CURVE('',#12686,#12687,#6709,.T.) ;
#15816=EDGE_CURVE('',#12687,#12688,#10918,.T.) ;
#15817=EDGE_CURVE('',#12688,#12689,#6710,.T.) ;
#15818=EDGE_CURVE('',#12689,#12686,#10919,.T.) ;
#15819=EDGE_CURVE('',#12690,#12691,#6711,.T.) ;
#15820=EDGE_CURVE('',#12690,#12692,#6712,.T.) ;
#15821=EDGE_CURVE('',#12692,#12693,#6713,.T.) ;
#15822=EDGE_CURVE('',#12693,#12691,#6714,.T.) ;
#15823=EDGE_CURVE('',#12689,#12693,#6715,.T.) ;
#15824=EDGE_CURVE('',#12692,#12694,#6716,.T.) ;
#15825=EDGE_CURVE('',#12694,#12695,#6717,.T.) ;
#15826=EDGE_CURVE('',#12695,#12686,#6718,.T.) ;
#15827=EDGE_CURVE('',#12694,#12696,#6719,.T.) ;
#15828=EDGE_CURVE('',#12696,#12697,#6720,.T.) ;
#15829=EDGE_CURVE('',#12697,#12695,#6721,.T.) ;
#15830=EDGE_CURVE('',#12691,#12688,#6722,.T.) ;
#15831=EDGE_CURVE('',#12696,#12690,#6723,.T.) ;
#15832=EDGE_CURVE('',#12687,#12697,#6724,.T.) ;
#15833=EDGE_CURVE('',#12698,#12698,#10920,.T.) ;
#15834=EDGE_CURVE('',#12698,#12699,#6725,.T.) ;
#15835=EDGE_CURVE('',#12699,#12699,#10921,.T.) ;
#15836=EDGE_CURVE('',#12700,#12700,#10922,.T.) ;
#15837=EDGE_CURVE('',#12700,#12701,#6726,.T.) ;
#15838=EDGE_CURVE('',#12701,#12701,#10923,.T.) ;
#15839=EDGE_CURVE('',#12702,#12703,#6727,.T.) ;
#15840=EDGE_CURVE('',#12703,#12704,#10924,.T.) ;
#15841=EDGE_CURVE('',#12704,#12705,#6728,.T.) ;
#15842=EDGE_CURVE('',#12705,#12702,#10925,.T.) ;
#15843=EDGE_CURVE('',#12706,#12707,#6729,.T.) ;
#15844=EDGE_CURVE('',#12706,#12708,#6730,.T.) ;
#15845=EDGE_CURVE('',#12708,#12709,#6731,.T.) ;
#15846=EDGE_CURVE('',#12709,#12707,#6732,.T.) ;
#15847=EDGE_CURVE('',#12705,#12709,#6733,.T.) ;
#15848=EDGE_CURVE('',#12708,#12710,#6734,.T.) ;
#15849=EDGE_CURVE('',#12710,#12711,#6735,.T.) ;
#15850=EDGE_CURVE('',#12711,#12702,#6736,.T.) ;
#15851=EDGE_CURVE('',#12710,#12712,#6737,.T.) ;
#15852=EDGE_CURVE('',#12712,#12713,#6738,.T.) ;
#15853=EDGE_CURVE('',#12713,#12711,#6739,.T.) ;
#15854=EDGE_CURVE('',#12707,#12704,#6740,.T.) ;
#15855=EDGE_CURVE('',#12712,#12706,#6741,.T.) ;
#15856=EDGE_CURVE('',#12703,#12713,#6742,.T.) ;
#15857=EDGE_CURVE('',#12714,#12714,#10926,.T.) ;
#15858=EDGE_CURVE('',#12714,#12715,#6743,.T.) ;
#15859=EDGE_CURVE('',#12715,#12715,#10927,.T.) ;
#15860=EDGE_CURVE('',#12716,#12716,#10928,.T.) ;
#15861=EDGE_CURVE('',#12716,#12717,#6744,.T.) ;
#15862=EDGE_CURVE('',#12717,#12717,#10929,.T.) ;
#15863=EDGE_CURVE('',#12718,#12718,#10930,.T.) ;
#15864=EDGE_CURVE('',#12718,#12719,#6745,.T.) ;
#15865=EDGE_CURVE('',#12719,#12719,#10931,.T.) ;
#15866=EDGE_CURVE('',#12720,#12720,#10932,.T.) ;
#15867=EDGE_CURVE('',#12720,#12721,#6746,.T.) ;
#15868=EDGE_CURVE('',#12721,#12721,#10933,.T.) ;
#15869=EDGE_CURVE('',#12722,#12723,#6747,.T.) ;
#15870=EDGE_CURVE('',#12723,#12724,#6748,.T.) ;
#15871=EDGE_CURVE('',#12724,#12725,#6749,.T.) ;
#15872=EDGE_CURVE('',#12726,#12725,#6750,.T.) ;
#15873=EDGE_CURVE('',#12726,#12722,#6751,.T.) ;
#15874=EDGE_CURVE('',#12727,#12727,#10934,.T.) ;
#15875=EDGE_CURVE('',#12728,#12728,#10935,.T.) ;
#15876=EDGE_CURVE('',#12728,#12729,#6752,.T.) ;
#15877=EDGE_CURVE('',#12729,#12729,#10936,.T.) ;
#15878=EDGE_CURVE('',#12730,#12730,#10937,.T.) ;
#15879=EDGE_CURVE('',#12730,#12727,#6753,.T.) ;
#15880=EDGE_CURVE('',#12731,#12732,#6754,.T.) ;
#15881=EDGE_CURVE('',#12731,#12733,#6755,.T.) ;
#15882=EDGE_CURVE('',#12734,#12733,#6756,.T.) ;
#15883=EDGE_CURVE('',#12732,#12734,#6757,.T.) ;
#15884=EDGE_CURVE('',#12732,#12735,#6758,.T.) ;
#15885=EDGE_CURVE('',#12736,#12734,#6759,.T.) ;
#15886=EDGE_CURVE('',#12735,#12736,#6760,.T.) ;
#15887=EDGE_CURVE('',#12735,#12737,#6761,.T.) ;
#15888=EDGE_CURVE('',#12738,#12736,#6762,.T.) ;
#15889=EDGE_CURVE('',#12737,#12738,#6763,.T.) ;
#15890=EDGE_CURVE('',#12737,#12731,#6764,.T.) ;
#15891=EDGE_CURVE('',#12733,#12738,#6765,.T.) ;
#15892=EDGE_CURVE('',#12739,#12740,#6766,.T.) ;
#15893=EDGE_CURVE('',#12740,#12741,#6767,.T.) ;
#15894=EDGE_CURVE('',#12741,#12742,#6768,.T.) ;
#15895=EDGE_CURVE('',#12742,#12739,#6769,.T.) ;
#15896=EDGE_CURVE('',#12743,#12742,#6770,.T.) ;
#15897=EDGE_CURVE('',#12744,#12741,#6771,.T.) ;
#15898=EDGE_CURVE('',#12743,#12744,#6772,.T.) ;
#15899=EDGE_CURVE('',#12745,#12740,#6773,.T.) ;
#15900=EDGE_CURVE('',#12746,#12739,#6774,.T.) ;
#15901=EDGE_CURVE('',#12745,#12746,#6775,.T.) ;
#15902=EDGE_CURVE('',#12744,#12747,#6776,.T.) ;
#15903=EDGE_CURVE('',#12748,#12747,#6777,.T.) ;
#15904=EDGE_CURVE('',#12749,#12748,#6778,.T.) ;
#15905=EDGE_CURVE('',#12749,#12743,#6779,.T.) ;
#15906=EDGE_CURVE('',#12750,#12751,#6780,.T.) ;
#15907=EDGE_CURVE('',#12750,#12752,#6781,.T.) ;
#15908=EDGE_CURVE('',#12752,#12753,#6782,.T.) ;
#15909=EDGE_CURVE('',#12751,#12753,#6783,.T.) ;
#15910=EDGE_CURVE('',#12754,#12754,#10938,.T.) ;
#15911=EDGE_CURVE('',#12755,#12756,#6784,.T.) ;
#15912=EDGE_CURVE('',#12756,#12757,#6785,.T.) ;
#15913=EDGE_CURVE('',#12757,#12758,#6786,.T.) ;
#15914=EDGE_CURVE('',#12758,#12755,#6787,.T.) ;
#15915=EDGE_CURVE('',#12759,#12750,#10939,.T.) ;
#15916=EDGE_CURVE('',#12760,#12759,#6788,.T.) ;
#15917=EDGE_CURVE('',#12760,#12761,#6789,.T.) ;
#15918=EDGE_CURVE('',#12762,#12761,#6790,.T.) ;
#15919=EDGE_CURVE('',#12755,#12762,#6791,.T.) ;
#15920=EDGE_CURVE('',#12763,#12758,#6792,.T.) ;
#15921=EDGE_CURVE('',#12764,#12763,#6793,.T.) ;
#15922=EDGE_CURVE('',#12764,#12752,#6794,.T.) ;
#15923=EDGE_CURVE('',#12765,#12766,#6795,.T.) ;
#15924=EDGE_CURVE('',#12767,#12765,#6796,.T.) ;
#15925=EDGE_CURVE('',#12767,#12757,#6797,.T.) ;
#15926=EDGE_CURVE('',#12756,#12768,#6798,.T.) ;
#15927=EDGE_CURVE('',#12769,#12768,#6799,.T.) ;
#15928=EDGE_CURVE('',#12770,#12769,#6800,.T.) ;
#15929=EDGE_CURVE('',#12766,#12770,#6801,.T.) ;
#15930=EDGE_CURVE('',#12763,#12767,#6802,.T.) ;
#15931=EDGE_CURVE('',#12766,#12771,#6803,.T.) ;
#15932=EDGE_CURVE('',#12771,#12772,#10940,.T.) ;
#15933=EDGE_CURVE('',#12772,#12773,#6804,.T.) ;
#15934=EDGE_CURVE('',#12766,#12773,#6805,.T.) ;
#15935=EDGE_CURVE('',#12753,#12774,#6806,.T.) ;
#15936=EDGE_CURVE('',#12774,#12775,#6807,.T.) ;
#15937=EDGE_CURVE('',#12775,#12751,#10941,.T.) ;
#15938=EDGE_CURVE('',#12776,#12772,#6808,.T.) ;
#15939=EDGE_CURVE('',#12777,#12776,#6809,.T.) ;
#15940=EDGE_CURVE('',#12777,#12773,#6810,.T.) ;
#15941=EDGE_CURVE('',#12778,#12779,#6811,.T.) ;
#15942=EDGE_CURVE('',#12780,#12778,#6812,.T.) ;
#15943=EDGE_CURVE('',#12781,#12780,#6813,.T.) ;
#15944=EDGE_CURVE('',#12779,#12781,#6814,.T.) ;
#15945=EDGE_CURVE('',#12782,#12783,#6815,.T.) ;
#15946=EDGE_CURVE('',#12784,#12782,#6816,.T.) ;
#15947=EDGE_CURVE('',#12785,#12784,#6817,.T.) ;
#15948=EDGE_CURVE('',#12783,#12785,#6818,.T.) ;
#15949=EDGE_CURVE('',#12786,#12787,#6819,.T.) ;
#15950=EDGE_CURVE('',#12786,#12788,#6820,.T.) ;
#15951=EDGE_CURVE('',#12789,#12788,#6821,.T.) ;
#15952=EDGE_CURVE('',#12789,#12787,#6822,.T.) ;
#15953=EDGE_CURVE('',#12774,#12790,#6823,.T.) ;
#15954=EDGE_CURVE('',#12791,#12790,#6824,.T.) ;
#15955=EDGE_CURVE('',#12775,#12791,#6825,.T.) ;
#15956=EDGE_CURVE('',#12792,#12793,#6826,.T.) ;
#15957=EDGE_CURVE('',#12794,#12792,#6827,.T.) ;
#15958=EDGE_CURVE('',#12794,#12795,#6828,.T.) ;
#15959=EDGE_CURVE('',#12795,#12793,#10942,.T.) ;
#15960=EDGE_CURVE('',#12795,#12796,#6829,.T.) ;
#15961=EDGE_CURVE('',#12797,#12796,#6830,.T.) ;
#15962=EDGE_CURVE('',#12793,#12797,#6831,.T.) ;
#15963=EDGE_CURVE('',#12793,#12795,#10943,.T.) ;
#15964=EDGE_CURVE('',#12798,#12799,#6832,.T.) ;
#15965=EDGE_CURVE('',#12800,#12799,#6833,.T.) ;
#15966=EDGE_CURVE('',#12800,#12801,#6834,.T.) ;
#15967=EDGE_CURVE('',#12801,#12802,#6835,.T.) ;
#15968=EDGE_CURVE('',#12802,#12803,#6836,.T.) ;
#15969=EDGE_CURVE('',#12792,#12803,#6837,.T.) ;
#15970=EDGE_CURVE('',#12804,#12797,#6838,.T.) ;
#15971=EDGE_CURVE('',#12787,#12804,#6839,.T.) ;
#15972=EDGE_CURVE('',#12789,#12805,#6840,.T.) ;
#15973=EDGE_CURVE('',#12806,#12805,#6841,.T.) ;
#15974=EDGE_CURVE('',#12807,#12806,#6842,.T.) ;
#15975=EDGE_CURVE('',#12808,#12807,#6843,.T.) ;
#15976=EDGE_CURVE('',#12809,#12808,#6844,.T.) ;
#15977=EDGE_CURVE('',#12809,#12810,#6845,.T.) ;
#15978=EDGE_CURVE('',#12810,#12798,#6846,.T.) ;
#15979=EDGE_CURVE('',#12811,#12812,#6847,.T.) ;
#15980=EDGE_CURVE('',#12813,#12811,#6848,.T.) ;
#15981=EDGE_CURVE('',#12813,#12725,#6849,.T.) ;
#15982=EDGE_CURVE('',#12724,#12814,#6850,.T.) ;
#15983=EDGE_CURVE('',#12815,#12814,#6851,.T.) ;
#15984=EDGE_CURVE('',#12815,#12790,#6852,.T.) ;
#15985=EDGE_CURVE('',#12812,#12764,#6853,.T.) ;
#15986=EDGE_CURVE('',#12807,#12816,#10944,.T.) ;
#15987=EDGE_CURVE('',#12817,#12816,#6854,.T.) ;
#15988=EDGE_CURVE('',#12808,#12817,#6855,.T.) ;
#15989=EDGE_CURVE('',#12818,#12804,#6856,.T.) ;
#15990=EDGE_CURVE('',#12786,#12818,#6857,.T.) ;
#15991=EDGE_CURVE('',#12788,#12819,#6858,.T.) ;
#15992=EDGE_CURVE('',#12805,#12819,#6859,.T.) ;
#15993=EDGE_CURVE('',#12785,#12820,#6860,.T.) ;
#15994=EDGE_CURVE('',#12821,#12820,#6861,.T.) ;
#15995=EDGE_CURVE('',#12783,#12821,#6862,.T.) ;
#15996=EDGE_CURVE('',#12822,#12821,#6863,.T.) ;
#15997=EDGE_CURVE('',#12782,#12822,#6864,.T.) ;
#15998=EDGE_CURVE('',#12781,#12823,#6865,.T.) ;
#15999=EDGE_CURVE('',#12824,#12823,#6866,.T.) ;
#16000=EDGE_CURVE('',#12779,#12824,#6867,.T.) ;
#16001=EDGE_CURVE('',#12825,#12824,#6868,.T.) ;
#16002=EDGE_CURVE('',#12778,#12825,#6869,.T.) ;
#16003=EDGE_CURVE('',#12796,#12818,#6870,.T.) ;
#16004=EDGE_CURVE('',#12820,#12826,#6871,.T.) ;
#16005=EDGE_CURVE('',#12826,#12822,#6872,.T.) ;
#16006=EDGE_CURVE('',#12803,#12827,#6873,.T.) ;
#16007=EDGE_CURVE('',#12827,#12794,#6874,.T.) ;
#16008=EDGE_CURVE('',#12828,#12828,#10945,.T.) ;
#16009=EDGE_CURVE('',#12829,#12829,#10946,.T.) ;
#16010=EDGE_CURVE('',#12819,#12830,#6875,.T.) ;
#16011=EDGE_CURVE('',#12830,#12806,#6876,.T.) ;
#16012=EDGE_CURVE('',#12823,#12831,#6877,.T.) ;
#16013=EDGE_CURVE('',#12831,#12825,#6878,.T.) ;
#16014=EDGE_CURVE('',#12832,#12811,#6879,.T.) ;
#16015=EDGE_CURVE('',#12832,#12833,#6880,.T.) ;
#16016=EDGE_CURVE('',#12813,#12833,#6881,.T.) ;
#16017=EDGE_CURVE('',#12812,#12765,#6882,.T.) ;
#16018=EDGE_CURVE('',#12832,#12765,#6883,.T.) ;
#16019=EDGE_CURVE('',#12816,#12830,#6884,.T.) ;
#16020=EDGE_CURVE('',#12816,#12807,#10947,.T.) ;
#16021=EDGE_CURVE('',#12784,#12826,#6885,.T.) ;
#16022=EDGE_CURVE('',#12780,#12831,#6886,.T.) ;
#16023=EDGE_CURVE('',#12834,#12834,#10948,.T.) ;
#16024=EDGE_CURVE('',#12835,#12835,#10949,.T.) ;
#16025=EDGE_CURVE('',#12836,#12836,#10950,.T.) ;
#16026=EDGE_CURVE('',#12837,#12837,#10951,.T.) ;
#16027=EDGE_CURVE('',#12807,#12836,#6887,.T.) ;
#16028=EDGE_CURVE('',#12834,#12793,#6888,.T.) ;
#16029=EDGE_CURVE('',#12837,#12829,#6889,.T.) ;
#16030=EDGE_CURVE('',#12828,#12835,#6890,.T.) ;
#16031=EDGE_CURVE('',#12799,#12838,#6891,.T.) ;
#16032=EDGE_CURVE('',#12838,#12839,#6892,.T.) ;
#16033=EDGE_CURVE('',#12839,#12800,#6893,.T.) ;
#16034=EDGE_CURVE('',#12840,#12841,#6894,.T.) ;
#16035=EDGE_CURVE('',#12842,#12841,#6895,.T.) ;
#16036=EDGE_CURVE('',#12843,#12842,#6896,.T.) ;
#16037=EDGE_CURVE('',#12840,#12843,#6897,.T.) ;
#16038=EDGE_CURVE('',#12844,#12845,#6898,.T.) ;
#16039=EDGE_CURVE('',#12846,#12845,#6899,.T.) ;
#16040=EDGE_CURVE('',#12847,#12846,#6900,.T.) ;
#16041=EDGE_CURVE('',#12844,#12847,#6901,.T.) ;
#16042=EDGE_CURVE('',#12843,#12844,#6902,.T.) ;
#16043=EDGE_CURVE('',#12847,#12840,#6903,.T.) ;
#16044=EDGE_CURVE('',#12848,#12849,#6904,.T.) ;
#16045=EDGE_CURVE('',#12848,#12842,#6905,.T.) ;
#16046=EDGE_CURVE('',#12841,#12849,#6906,.T.) ;
#16047=EDGE_CURVE('',#12801,#12846,#6907,.T.) ;
#16048=EDGE_CURVE('',#12845,#12802,#6908,.T.) ;
#16049=EDGE_CURVE('',#12849,#12839,#6909,.T.) ;
#16050=EDGE_CURVE('',#12827,#12848,#6910,.T.) ;
#16051=EDGE_CURVE('',#12850,#12851,#6911,.T.) ;
#16052=EDGE_CURVE('',#12851,#12852,#6912,.T.) ;
#16053=EDGE_CURVE('',#12852,#12853,#6913,.T.) ;
#16054=EDGE_CURVE('',#12853,#12850,#6914,.T.) ;
#16055=EDGE_CURVE('',#12770,#12760,#6915,.T.) ;
#16056=EDGE_CURVE('',#12771,#12759,#6916,.T.) ;
#16057=EDGE_CURVE('',#12768,#12762,#6917,.T.) ;
#16058=EDGE_CURVE('',#12761,#12769,#6918,.T.) ;
#16059=EDGE_CURVE('',#12854,#12855,#6919,.T.) ;
#16060=EDGE_CURVE('',#12855,#12856,#6920,.T.) ;
#16061=EDGE_CURVE('',#12856,#12857,#6921,.T.) ;
#16062=EDGE_CURVE('',#12857,#12854,#6922,.T.) ;
#16063=EDGE_CURVE('',#12853,#12854,#6923,.T.) ;
#16064=EDGE_CURVE('',#12850,#12857,#6924,.T.) ;
#16065=EDGE_CURVE('',#12852,#12855,#6925,.T.) ;
#16066=EDGE_CURVE('',#12851,#12856,#6926,.T.) ;
#16067=EDGE_CURVE('',#12858,#12858,#10952,.T.) ;
#16068=EDGE_CURVE('',#12859,#12859,#10953,.T.) ;
#16069=EDGE_CURVE('',#12860,#12860,#10954,.T.) ;
#16070=EDGE_CURVE('',#12859,#12861,#6927,.T.) ;
#16071=EDGE_CURVE('',#12861,#12861,#10955,.T.) ;
#16072=EDGE_CURVE('',#12754,#12860,#6928,.T.) ;
#16073=EDGE_CURVE('',#12862,#12862,#10956,.T.) ;
#16074=EDGE_CURVE('',#12863,#12863,#10957,.T.) ;
#16075=EDGE_CURVE('',#12864,#12864,#10958,.T.) ;
#16076=EDGE_CURVE('',#12863,#12862,#6929,.T.) ;
#16077=EDGE_CURVE('',#12858,#12864,#6930,.T.) ;
#16078=EDGE_CURVE('',#12865,#12866,#6931,.T.) ;
#16079=EDGE_CURVE('',#12866,#12749,#10959,.T.) ;
#16080=EDGE_CURVE('',#12776,#12748,#10960,.T.) ;
#16081=EDGE_CURVE('',#12865,#12791,#10961,.T.) ;
#16082=EDGE_CURVE('',#12815,#12865,#6932,.T.) ;
#16083=EDGE_CURVE('',#12833,#12726,#6933,.T.) ;
#16084=EDGE_CURVE('',#12747,#12777,#6934,.T.) ;
#16085=EDGE_CURVE('',#12722,#12867,#6935,.T.) ;
#16086=EDGE_CURVE('',#12868,#12867,#6936,.T.) ;
#16087=EDGE_CURVE('',#12723,#12868,#6937,.T.) ;
#16088=EDGE_CURVE('',#12814,#12866,#6938,.T.) ;
#16089=EDGE_CURVE('',#12746,#12868,#6939,.T.) ;
#16090=EDGE_CURVE('',#12867,#12745,#6940,.T.) ;
#16091=EDGE_CURVE('',#12726,#12747,#6941,.T.) ;
#16092=EDGE_CURVE('',#12869,#12809,#6942,.T.) ;
#16093=EDGE_CURVE('',#12817,#12869,#6943,.T.) ;
#16094=EDGE_CURVE('',#12838,#12870,#6944,.T.) ;
#16095=EDGE_CURVE('',#12870,#12871,#6945,.T.) ;
#16096=EDGE_CURVE('',#12871,#12869,#6946,.T.) ;
#16097=EDGE_CURVE('',#12872,#12873,#6947,.T.) ;
#16098=EDGE_CURVE('',#12874,#12873,#6948,.T.) ;
#16099=EDGE_CURVE('',#12875,#12874,#6949,.T.) ;
#16100=EDGE_CURVE('',#12872,#12875,#6950,.T.) ;
#16101=EDGE_CURVE('',#12876,#12877,#6951,.T.) ;
#16102=EDGE_CURVE('',#12878,#12877,#6952,.T.) ;
#16103=EDGE_CURVE('',#12879,#12878,#6953,.T.) ;
#16104=EDGE_CURVE('',#12876,#12879,#6954,.T.) ;
#16105=EDGE_CURVE('',#12873,#12871,#6955,.T.) ;
#16106=EDGE_CURVE('',#12879,#12872,#6956,.T.) ;
#16107=EDGE_CURVE('',#12810,#12878,#6957,.T.) ;
#16108=EDGE_CURVE('',#12870,#12874,#6958,.T.) ;
#16109=EDGE_CURVE('',#12875,#12876,#6959,.T.) ;
#16110=EDGE_CURVE('',#12877,#12798,#6960,.T.) ;
#16111=EDGE_CURVE('',#12880,#12881,#10962,.T.) ;
#16112=EDGE_CURVE('',#12882,#12880,#6961,.T.) ;
#16113=EDGE_CURVE('',#12883,#12882,#10963,.T.) ;
#16114=EDGE_CURVE('',#12881,#12883,#6962,.T.) ;
#16115=EDGE_CURVE('',#12884,#12883,#6963,.T.) ;
#16116=EDGE_CURVE('',#12884,#12885,#6964,.T.) ;
#16117=EDGE_CURVE('',#12885,#12881,#6965,.T.) ;
#16118=EDGE_CURVE('',#12886,#12882,#6966,.T.) ;
#16119=EDGE_CURVE('',#12886,#12884,#6967,.T.) ;
#16120=EDGE_CURVE('',#12887,#12880,#6968,.T.) ;
#16121=EDGE_CURVE('',#12887,#12886,#6969,.T.) ;
#16122=EDGE_CURVE('',#12885,#12887,#6970,.T.) ;
#16123=EDGE_CURVE('',#12888,#12889,#6971,.T.) ;
#16124=EDGE_CURVE('',#12890,#12888,#6972,.T.) ;
#16125=EDGE_CURVE('',#12891,#12890,#6973,.T.) ;
#16126=EDGE_CURVE('',#12889,#12891,#6974,.T.) ;
#16127=EDGE_CURVE('',#12892,#12893,#10964,.T.) ;
#16128=EDGE_CURVE('',#12891,#12893,#6975,.T.) ;
#16129=EDGE_CURVE('',#12890,#12892,#6976,.T.) ;
#16130=EDGE_CURVE('',#12894,#12892,#6977,.T.) ;
#16131=EDGE_CURVE('',#12888,#12894,#6978,.T.) ;
#16132=EDGE_CURVE('',#12895,#12894,#10965,.T.) ;
#16133=EDGE_CURVE('',#12889,#12895,#6979,.T.) ;
#16134=EDGE_CURVE('',#12893,#12895,#6980,.T.) ;
#16135=EDGE_CURVE('',#12896,#12897,#10966,.T.) ;
#16136=EDGE_CURVE('',#12896,#12897,#6981,.T.) ;
#16137=EDGE_CURVE('',#12898,#12899,#10967,.T.) ;
#16138=EDGE_CURVE('',#12898,#12899,#6982,.T.) ;
#16139=EDGE_CURVE('',#12897,#12898,#6983,.T.) ;
#16140=EDGE_CURVE('',#12899,#12896,#6984,.T.) ;
#16141=EDGE_CURVE('',#12900,#12901,#6985,.T.) ;
#16142=EDGE_CURVE('',#12902,#12900,#6986,.T.) ;
#16143=EDGE_CURVE('',#12903,#12902,#6987,.T.) ;
#16144=EDGE_CURVE('',#12901,#12903,#6988,.T.) ;
#16145=EDGE_CURVE('',#12901,#12904,#6989,.T.) ;
#16146=EDGE_CURVE('',#12905,#12903,#6990,.T.) ;
#16147=EDGE_CURVE('',#12904,#12905,#6991,.T.) ;
#16148=EDGE_CURVE('',#12904,#12900,#10968,.T.) ;
#16149=EDGE_CURVE('',#12902,#12905,#10969,.T.) ;
#16150=EDGE_CURVE('',#12906,#12907,#6992,.T.) ;
#16151=EDGE_CURVE('',#12907,#12908,#10970,.T.) ;
#16152=EDGE_CURVE('',#12908,#12906,#6993,.T.) ;
#16153=EDGE_CURVE('',#12909,#12906,#6994,.T.) ;
#16154=EDGE_CURVE('',#12908,#12910,#6995,.T.) ;
#16155=EDGE_CURVE('',#12910,#12909,#6996,.T.) ;
#16156=EDGE_CURVE('',#12911,#12909,#6997,.T.) ;
#16157=EDGE_CURVE('',#12910,#12911,#10971,.T.) ;
#16158=EDGE_CURVE('',#12907,#12911,#6998,.T.) ;
#16159=EDGE_CURVE('',#12912,#12913,#6999,.T.) ;
#16160=EDGE_CURVE('',#12914,#12912,#7000,.T.) ;
#16161=EDGE_CURVE('',#12915,#12914,#7001,.T.) ;
#16162=EDGE_CURVE('',#12913,#12915,#7002,.T.) ;
#16163=EDGE_CURVE('',#12916,#12912,#7003,.T.) ;
#16164=EDGE_CURVE('',#12917,#12916,#7004,.T.) ;
#16165=EDGE_CURVE('',#12914,#12917,#7005,.T.) ;
#16166=EDGE_CURVE('',#12913,#12916,#10972,.T.) ;
#16167=EDGE_CURVE('',#12917,#12915,#10973,.T.) ;
#16168=EDGE_CURVE('',#12918,#12919,#7006,.T.) ;
#16169=EDGE_CURVE('',#12920,#12919,#7007,.T.) ;
#16170=EDGE_CURVE('',#12920,#12918,#10974,.T.) ;
#16171=EDGE_CURVE('',#12921,#12922,#7008,.T.) ;
#16172=EDGE_CURVE('',#12922,#12923,#10975,.T.) ;
#16173=EDGE_CURVE('',#12923,#12921,#7009,.T.) ;
#16174=EDGE_CURVE('',#12922,#12918,#7010,.T.) ;
#16175=EDGE_CURVE('',#12923,#12920,#7011,.T.) ;
#16176=EDGE_CURVE('',#12919,#12921,#7012,.T.) ;
#16177=EDGE_CURVE('',#12924,#12925,#7013,.T.) ;
#16178=EDGE_CURVE('',#12926,#12924,#7014,.T.) ;
#16179=EDGE_CURVE('',#12927,#12926,#7015,.T.) ;
#16180=EDGE_CURVE('',#12925,#12927,#7016,.T.) ;
#16181=EDGE_CURVE('',#12928,#12924,#10976,.T.) ;
#16182=EDGE_CURVE('',#12929,#12928,#7017,.T.) ;
#16183=EDGE_CURVE('',#12926,#12929,#10977,.T.) ;
#16184=EDGE_CURVE('',#12928,#12925,#7018,.T.) ;
#16185=EDGE_CURVE('',#12929,#12927,#7019,.T.) ;
#16186=EDGE_CURVE('',#12930,#12931,#7020,.T.) ;
#16187=EDGE_CURVE('',#12932,#12931,#7021,.T.) ;
#16188=EDGE_CURVE('',#12932,#12930,#10978,.T.) ;
#16189=EDGE_CURVE('',#12933,#12934,#7022,.T.) ;
#16190=EDGE_CURVE('',#12934,#12935,#10979,.T.) ;
#16191=EDGE_CURVE('',#12935,#12933,#7023,.T.) ;
#16192=EDGE_CURVE('',#12934,#12930,#7024,.T.) ;
#16193=EDGE_CURVE('',#12935,#12932,#7025,.T.) ;
#16194=EDGE_CURVE('',#12931,#12933,#7026,.T.) ;
#16195=EDGE_CURVE('',#12936,#12937,#7027,.T.) ;
#16196=EDGE_CURVE('',#12938,#12936,#7028,.T.) ;
#16197=EDGE_CURVE('',#12939,#12938,#7029,.T.) ;
#16198=EDGE_CURVE('',#12937,#12939,#7030,.T.) ;
#16199=EDGE_CURVE('',#12939,#12937,#10980,.T.) ;
#16200=EDGE_CURVE('',#12936,#12938,#10981,.T.) ;
#16201=EDGE_CURVE('',#12940,#12941,#7031,.T.) ;
#16202=EDGE_CURVE('',#12942,#12941,#10982,.T.) ;
#16203=EDGE_CURVE('',#12942,#12943,#7032,.T.) ;
#16204=EDGE_CURVE('',#12940,#12943,#10983,.T.) ;
#16205=EDGE_CURVE('',#12943,#12940,#7033,.T.) ;
#16206=EDGE_CURVE('',#12941,#12942,#7034,.T.) ;
#16207=EDGE_CURVE('',#12944,#12945,#7035,.T.) ;
#16208=EDGE_CURVE('',#12946,#12944,#7036,.T.) ;
#16209=EDGE_CURVE('',#12947,#12946,#7037,.T.) ;
#16210=EDGE_CURVE('',#12945,#12947,#7038,.T.) ;
#16211=EDGE_CURVE('',#12946,#12947,#10984,.T.) ;
#16212=EDGE_CURVE('',#12945,#12944,#10985,.T.) ;
#16213=EDGE_CURVE('',#12948,#12949,#7039,.T.) ;
#16214=EDGE_CURVE('',#12950,#12949,#10986,.T.) ;
#16215=EDGE_CURVE('',#12950,#12951,#7040,.T.) ;
#16216=EDGE_CURVE('',#12948,#12951,#10987,.T.) ;
#16217=EDGE_CURVE('',#12949,#12950,#7041,.T.) ;
#16218=EDGE_CURVE('',#12951,#12948,#7042,.T.) ;
#16219=EDGE_CURVE('',#12952,#12953,#7043,.T.) ;
#16220=EDGE_CURVE('',#12954,#12952,#7044,.T.) ;
#16221=EDGE_CURVE('',#12955,#12954,#7045,.T.) ;
#16222=EDGE_CURVE('',#12953,#12955,#7046,.T.) ;
#16223=EDGE_CURVE('',#12952,#12954,#10988,.T.) ;
#16224=EDGE_CURVE('',#12955,#12953,#10989,.T.) ;
#16225=EDGE_CURVE('',#12956,#12957,#7047,.T.) ;
#16226=EDGE_CURVE('',#12957,#12958,#7048,.T.) ;
#16227=EDGE_CURVE('',#12958,#12959,#7049,.T.) ;
#16228=EDGE_CURVE('',#12956,#12959,#7050,.T.) ;
#16229=EDGE_CURVE('',#12957,#12960,#7051,.T.) ;
#16230=EDGE_CURVE('',#12960,#12961,#7052,.T.) ;
#16231=EDGE_CURVE('',#12961,#12958,#7053,.T.) ;
#16232=EDGE_CURVE('',#12962,#12956,#7054,.T.) ;
#16233=EDGE_CURVE('',#12959,#12963,#7055,.T.) ;
#16234=EDGE_CURVE('',#12962,#12963,#7056,.T.) ;
#16235=EDGE_CURVE('',#12960,#12962,#7057,.T.) ;
#16236=EDGE_CURVE('',#12963,#12961,#7058,.T.) ;
#16237=EDGE_CURVE('',#12964,#12965,#7059,.T.) ;
#16238=EDGE_CURVE('',#12966,#12964,#7060,.T.) ;
#16239=EDGE_CURVE('',#12967,#12966,#7061,.T.) ;
#16240=EDGE_CURVE('',#12965,#12967,#7062,.T.) ;
#16241=EDGE_CURVE('',#12968,#12969,#7063,.T.) ;
#16242=EDGE_CURVE('',#12970,#12968,#7064,.T.) ;
#16243=EDGE_CURVE('',#12971,#12970,#7065,.T.) ;
#16244=EDGE_CURVE('',#12969,#12971,#7066,.T.) ;
#16245=EDGE_CURVE('',#12965,#12968,#7067,.T.) ;
#16246=EDGE_CURVE('',#12964,#12969,#7068,.T.) ;
#16247=EDGE_CURVE('',#12967,#12970,#7069,.T.) ;
#16248=EDGE_CURVE('',#12966,#12971,#7070,.T.) ;
#16249=EDGE_CURVE('',#12972,#12973,#7071,.T.) ;
#16250=EDGE_CURVE('',#12974,#12972,#7072,.T.) ;
#16251=EDGE_CURVE('',#12975,#12974,#7073,.T.) ;
#16252=EDGE_CURVE('',#12973,#12975,#7074,.T.) ;
#16253=EDGE_CURVE('',#12976,#12972,#7075,.T.) ;
#16254=EDGE_CURVE('',#12976,#12977,#7076,.T.) ;
#16255=EDGE_CURVE('',#12974,#12977,#7077,.T.) ;
#16256=EDGE_CURVE('',#12978,#12976,#7078,.T.) ;
#16257=EDGE_CURVE('',#12979,#12978,#7079,.T.) ;
#16258=EDGE_CURVE('',#12977,#12979,#7080,.T.) ;
#16259=EDGE_CURVE('',#12979,#12980,#7081,.T.) ;
#16260=EDGE_CURVE('',#12980,#12981,#7082,.T.) ;
#16261=EDGE_CURVE('',#12981,#12982,#7083,.T.) ;
#16262=EDGE_CURVE('',#12982,#12983,#7084,.T.) ;
#16263=EDGE_CURVE('',#12983,#12984,#7085,.T.) ;
#16264=EDGE_CURVE('',#12985,#12984,#7086,.T.) ;
#16265=EDGE_CURVE('',#12985,#12986,#7087,.T.) ;
#16266=EDGE_CURVE('',#12987,#12986,#7088,.T.) ;
#16267=EDGE_CURVE('',#12987,#12975,#7089,.T.) ;
#16268=EDGE_CURVE('',#12988,#12978,#7090,.T.) ;
#16269=EDGE_CURVE('',#12988,#12980,#7091,.T.) ;
#16270=EDGE_CURVE('',#12989,#12987,#7092,.T.) ;
#16271=EDGE_CURVE('',#12973,#12989,#7093,.T.) ;
#16272=EDGE_CURVE('',#12990,#12989,#7094,.T.) ;
#16273=EDGE_CURVE('',#12990,#12991,#7095,.T.) ;
#16274=EDGE_CURVE('',#12992,#12991,#7096,.T.) ;
#16275=EDGE_CURVE('',#12992,#12993,#7097,.T.) ;
#16276=EDGE_CURVE('',#12993,#12994,#7098,.T.) ;
#16277=EDGE_CURVE('',#12994,#12995,#7099,.T.) ;
#16278=EDGE_CURVE('',#12995,#12988,#7100,.T.) ;
#16279=EDGE_CURVE('',#12991,#12985,#7101,.T.) ;
#16280=EDGE_CURVE('',#12986,#12990,#7102,.T.) ;
#16281=EDGE_CURVE('',#12984,#12992,#7103,.T.) ;
#16282=EDGE_CURVE('',#12983,#12993,#7104,.T.) ;
#16283=EDGE_CURVE('',#12994,#12982,#7105,.T.) ;
#16284=EDGE_CURVE('',#12981,#12995,#7106,.T.) ;
#16285=EDGE_CURVE('',#12996,#12997,#7107,.T.) ;
#16286=EDGE_CURVE('',#12997,#12998,#10990,.T.) ;
#16287=EDGE_CURVE('',#12998,#12999,#7108,.T.) ;
#16288=EDGE_CURVE('',#12999,#12996,#10991,.T.) ;
#16289=EDGE_CURVE('',#12997,#12998,#7109,.T.) ;
#16290=EDGE_CURVE('',#12999,#12996,#7110,.T.) ;
#16291=EDGE_CURVE('',#13000,#13001,#10992,.T.) ;
#16292=EDGE_CURVE('',#13001,#13000,#7111,.T.) ;
#16293=EDGE_CURVE('',#13002,#13000,#7112,.T.) ;
#16294=EDGE_CURVE('',#13003,#13002,#7113,.T.) ;
#16295=EDGE_CURVE('',#13001,#13003,#7114,.T.) ;
#16296=EDGE_CURVE('',#13004,#13003,#10993,.T.) ;
#16297=EDGE_CURVE('',#13004,#13005,#7115,.T.) ;
#16298=EDGE_CURVE('',#13006,#13005,#10994,.T.) ;
#16299=EDGE_CURVE('',#13006,#13007,#7116,.T.) ;
#16300=EDGE_CURVE('',#13007,#13008,#10995,.T.) ;
#16301=EDGE_CURVE('',#13008,#13009,#7117,.T.) ;
#16302=EDGE_CURVE('',#13010,#13009,#10996,.T.) ;
#16303=EDGE_CURVE('',#13010,#13011,#7118,.T.) ;
#16304=EDGE_CURVE('',#13002,#13011,#10997,.T.) ;
#16305=EDGE_CURVE('',#13008,#13007,#7119,.T.) ;
#16306=EDGE_CURVE('',#13009,#13006,#7120,.T.) ;
#16307=EDGE_CURVE('',#13005,#13010,#7121,.T.) ;
#16308=EDGE_CURVE('',#13011,#13004,#7122,.T.) ;
#21063=ORIENTED_EDGE('',*,*,#15797,.F.) ;
#21064=ORIENTED_EDGE('',*,*,#15798,.T.) ;
#21065=ORIENTED_EDGE('',*,*,#15799,.F.) ;
#21066=ORIENTED_EDGE('',*,*,#15798,.F.) ;
#21067=ORIENTED_EDGE('',*,*,#15800,.F.) ;
#21068=ORIENTED_EDGE('',*,*,#15801,.T.) ;
#21069=ORIENTED_EDGE('',*,*,#15802,.F.) ;
#21070=ORIENTED_EDGE('',*,*,#15801,.F.) ;
#21071=ORIENTED_EDGE('',*,*,#15803,.F.) ;
#21072=ORIENTED_EDGE('',*,*,#15804,.T.) ;
#21073=ORIENTED_EDGE('',*,*,#15805,.F.) ;
#21074=ORIENTED_EDGE('',*,*,#15804,.F.) ;
#21075=ORIENTED_EDGE('',*,*,#15806,.F.) ;
#21076=ORIENTED_EDGE('',*,*,#15807,.T.) ;
#21077=ORIENTED_EDGE('',*,*,#15808,.F.) ;
#21078=ORIENTED_EDGE('',*,*,#15807,.F.) ;
#21079=ORIENTED_EDGE('',*,*,#15809,.F.) ;
#21080=ORIENTED_EDGE('',*,*,#15810,.T.) ;
#21081=ORIENTED_EDGE('',*,*,#15811,.F.) ;
#21082=ORIENTED_EDGE('',*,*,#15810,.F.) ;
#21083=ORIENTED_EDGE('',*,*,#15812,.F.) ;
#21084=ORIENTED_EDGE('',*,*,#15813,.T.) ;
#21085=ORIENTED_EDGE('',*,*,#15814,.F.) ;
#21086=ORIENTED_EDGE('',*,*,#15813,.F.) ;
#21087=ORIENTED_EDGE('',*,*,#15815,.T.) ;
#21088=ORIENTED_EDGE('',*,*,#15816,.T.) ;
#21089=ORIENTED_EDGE('',*,*,#15817,.T.) ;
#21090=ORIENTED_EDGE('',*,*,#15818,.T.) ;
#21091=ORIENTED_EDGE('',*,*,#15819,.F.) ;
#21092=ORIENTED_EDGE('',*,*,#15820,.T.) ;
#21093=ORIENTED_EDGE('',*,*,#15821,.T.) ;
#21094=ORIENTED_EDGE('',*,*,#15822,.T.) ;
#21095=ORIENTED_EDGE('',*,*,#15818,.F.) ;
#21096=ORIENTED_EDGE('',*,*,#15823,.T.) ;
#21097=ORIENTED_EDGE('',*,*,#15821,.F.) ;
#21098=ORIENTED_EDGE('',*,*,#15824,.T.) ;
#21099=ORIENTED_EDGE('',*,*,#15825,.T.) ;
#21100=ORIENTED_EDGE('',*,*,#15826,.T.) ;
#21101=ORIENTED_EDGE('',*,*,#15825,.F.) ;
#21102=ORIENTED_EDGE('',*,*,#15827,.T.) ;
#21103=ORIENTED_EDGE('',*,*,#15828,.T.) ;
#21104=ORIENTED_EDGE('',*,*,#15829,.T.) ;
#21105=ORIENTED_EDGE('',*,*,#15817,.F.) ;
#21106=ORIENTED_EDGE('',*,*,#15830,.F.) ;
#21107=ORIENTED_EDGE('',*,*,#15822,.F.) ;
#21108=ORIENTED_EDGE('',*,*,#15823,.F.) ;
#21109=ORIENTED_EDGE('',*,*,#15802,.T.) ;
#21110=ORIENTED_EDGE('',*,*,#15814,.T.) ;
#21111=ORIENTED_EDGE('',*,*,#15820,.F.) ;
#21112=ORIENTED_EDGE('',*,*,#15831,.F.) ;
#21113=ORIENTED_EDGE('',*,*,#15827,.F.) ;
#21114=ORIENTED_EDGE('',*,*,#15824,.F.) ;
#21115=ORIENTED_EDGE('',*,*,#15797,.T.) ;
#21116=ORIENTED_EDGE('',*,*,#15809,.T.) ;
#21117=ORIENTED_EDGE('',*,*,#15815,.F.) ;
#21118=ORIENTED_EDGE('',*,*,#15826,.F.) ;
#21119=ORIENTED_EDGE('',*,*,#15829,.F.) ;
#21120=ORIENTED_EDGE('',*,*,#15832,.F.) ;
#21121=ORIENTED_EDGE('',*,*,#15816,.F.) ;
#21122=ORIENTED_EDGE('',*,*,#15832,.T.) ;
#21123=ORIENTED_EDGE('',*,*,#15828,.F.) ;
#21124=ORIENTED_EDGE('',*,*,#15831,.T.) ;
#21125=ORIENTED_EDGE('',*,*,#15819,.T.) ;
#21126=ORIENTED_EDGE('',*,*,#15830,.T.) ;
#21127=ORIENTED_EDGE('',*,*,#15833,.F.) ;
#21128=ORIENTED_EDGE('',*,*,#15834,.T.) ;
#21129=ORIENTED_EDGE('',*,*,#15835,.F.) ;
#21130=ORIENTED_EDGE('',*,*,#15834,.F.) ;
#21131=ORIENTED_EDGE('',*,*,#15836,.F.) ;
#21132=ORIENTED_EDGE('',*,*,#15837,.T.) ;
#21133=ORIENTED_EDGE('',*,*,#15838,.F.) ;
#21134=ORIENTED_EDGE('',*,*,#15837,.F.) ;
#21135=ORIENTED_EDGE('',*,*,#15839,.T.) ;
#21136=ORIENTED_EDGE('',*,*,#15840,.T.) ;
#21137=ORIENTED_EDGE('',*,*,#15841,.T.) ;
#21138=ORIENTED_EDGE('',*,*,#15842,.T.) ;
#21139=ORIENTED_EDGE('',*,*,#15843,.F.) ;
#21140=ORIENTED_EDGE('',*,*,#15844,.T.) ;
#21141=ORIENTED_EDGE('',*,*,#15845,.T.) ;
#21142=ORIENTED_EDGE('',*,*,#15846,.T.) ;
#21143=ORIENTED_EDGE('',*,*,#15842,.F.) ;
#21144=ORIENTED_EDGE('',*,*,#15847,.T.) ;
#21145=ORIENTED_EDGE('',*,*,#15845,.F.) ;
#21146=ORIENTED_EDGE('',*,*,#15848,.T.) ;
#21147=ORIENTED_EDGE('',*,*,#15849,.T.) ;
#21148=ORIENTED_EDGE('',*,*,#15850,.T.) ;
#21149=ORIENTED_EDGE('',*,*,#15849,.F.) ;
#21150=ORIENTED_EDGE('',*,*,#15851,.T.) ;
#21151=ORIENTED_EDGE('',*,*,#15852,.T.) ;
#21152=ORIENTED_EDGE('',*,*,#15853,.T.) ;
#21153=ORIENTED_EDGE('',*,*,#15841,.F.) ;
#21154=ORIENTED_EDGE('',*,*,#15854,.F.) ;
#21155=ORIENTED_EDGE('',*,*,#15846,.F.) ;
#21156=ORIENTED_EDGE('',*,*,#15847,.F.) ;
#21157=ORIENTED_EDGE('',*,*,#15808,.T.) ;
#21158=ORIENTED_EDGE('',*,*,#15838,.T.) ;
#21159=ORIENTED_EDGE('',*,*,#15844,.F.) ;
#21160=ORIENTED_EDGE('',*,*,#15855,.F.) ;
#21161=ORIENTED_EDGE('',*,*,#15851,.F.) ;
#21162=ORIENTED_EDGE('',*,*,#15848,.F.) ;
#21163=ORIENTED_EDGE('',*,*,#15803,.T.) ;
#21164=ORIENTED_EDGE('',*,*,#15833,.T.) ;
#21165=ORIENTED_EDGE('',*,*,#15839,.F.) ;
#21166=ORIENTED_EDGE('',*,*,#15850,.F.) ;
#21167=ORIENTED_EDGE('',*,*,#15853,.F.) ;
#21168=ORIENTED_EDGE('',*,*,#15856,.F.) ;
#21169=ORIENTED_EDGE('',*,*,#15840,.F.) ;
#21170=ORIENTED_EDGE('',*,*,#15856,.T.) ;
#21171=ORIENTED_EDGE('',*,*,#15852,.F.) ;
#21172=ORIENTED_EDGE('',*,*,#15855,.T.) ;
#21173=ORIENTED_EDGE('',*,*,#15843,.T.) ;
#21174=ORIENTED_EDGE('',*,*,#15854,.T.) ;
#21175=ORIENTED_EDGE('',*,*,#15857,.F.) ;
#21176=ORIENTED_EDGE('',*,*,#15858,.T.) ;
#21177=ORIENTED_EDGE('',*,*,#15859,.F.) ;
#21178=ORIENTED_EDGE('',*,*,#15858,.F.) ;
#21179=ORIENTED_EDGE('',*,*,#15860,.F.) ;
#21180=ORIENTED_EDGE('',*,*,#15861,.T.) ;
#21181=ORIENTED_EDGE('',*,*,#15862,.F.) ;
#21182=ORIENTED_EDGE('',*,*,#15861,.F.) ;
#21183=ORIENTED_EDGE('',*,*,#15863,.F.) ;
#21184=ORIENTED_EDGE('',*,*,#15864,.T.) ;
#21185=ORIENTED_EDGE('',*,*,#15865,.F.) ;
#21186=ORIENTED_EDGE('',*,*,#15864,.F.) ;
#21187=ORIENTED_EDGE('',*,*,#15866,.F.) ;
#21188=ORIENTED_EDGE('',*,*,#15867,.T.) ;
#21189=ORIENTED_EDGE('',*,*,#15868,.F.) ;
#21190=ORIENTED_EDGE('',*,*,#15867,.F.) ;
#21191=ORIENTED_EDGE('',*,*,#15866,.T.) ;
#21192=ORIENTED_EDGE('',*,*,#15865,.T.) ;
#21193=ORIENTED_EDGE('',*,*,#15869,.T.) ;
#21194=ORIENTED_EDGE('',*,*,#15870,.T.) ;
#21195=ORIENTED_EDGE('',*,*,#15871,.T.) ;
#21196=ORIENTED_EDGE('',*,*,#15872,.F.) ;
#21197=ORIENTED_EDGE('',*,*,#15873,.T.) ;
#21198=ORIENTED_EDGE('',*,*,#15799,.T.) ;
#21199=ORIENTED_EDGE('',*,*,#15811,.T.) ;
#21200=ORIENTED_EDGE('',*,*,#15874,.T.) ;
#21201=ORIENTED_EDGE('',*,*,#15868,.T.) ;
#21202=ORIENTED_EDGE('',*,*,#15875,.F.) ;
#21203=ORIENTED_EDGE('',*,*,#15876,.T.) ;
#21204=ORIENTED_EDGE('',*,*,#15877,.F.) ;
#21205=ORIENTED_EDGE('',*,*,#15876,.F.) ;
#21206=ORIENTED_EDGE('',*,*,#15878,.F.) ;
#21207=ORIENTED_EDGE('',*,*,#15879,.T.) ;
#21208=ORIENTED_EDGE('',*,*,#15874,.F.) ;
#21209=ORIENTED_EDGE('',*,*,#15879,.F.) ;
#21210=ORIENTED_EDGE('',*,*,#15878,.T.) ;
#21211=ORIENTED_EDGE('',*,*,#15877,.T.) ;
#21212=ORIENTED_EDGE('',*,*,#15863,.T.) ;
#21213=ORIENTED_EDGE('',*,*,#15880,.F.) ;
#21214=ORIENTED_EDGE('',*,*,#15881,.T.) ;
#21215=ORIENTED_EDGE('',*,*,#15882,.F.) ;
#21216=ORIENTED_EDGE('',*,*,#15883,.F.) ;
#21217=ORIENTED_EDGE('',*,*,#15884,.F.) ;
#21218=ORIENTED_EDGE('',*,*,#15883,.T.) ;
#21219=ORIENTED_EDGE('',*,*,#15885,.F.) ;
#21220=ORIENTED_EDGE('',*,*,#15886,.F.) ;
#21221=ORIENTED_EDGE('',*,*,#15887,.F.) ;
#21222=ORIENTED_EDGE('',*,*,#15886,.T.) ;
#21223=ORIENTED_EDGE('',*,*,#15888,.F.) ;
#21224=ORIENTED_EDGE('',*,*,#15889,.F.) ;
#21225=ORIENTED_EDGE('',*,*,#15890,.F.) ;
#21226=ORIENTED_EDGE('',*,*,#15889,.T.) ;
#21227=ORIENTED_EDGE('',*,*,#15891,.F.) ;
#21228=ORIENTED_EDGE('',*,*,#15881,.F.) ;
#21229=ORIENTED_EDGE('',*,*,#15892,.T.) ;
#21230=ORIENTED_EDGE('',*,*,#15893,.T.) ;
#21231=ORIENTED_EDGE('',*,*,#15894,.T.) ;
#21232=ORIENTED_EDGE('',*,*,#15895,.T.) ;
#21233=ORIENTED_EDGE('',*,*,#15888,.T.) ;
#21234=ORIENTED_EDGE('',*,*,#15885,.T.) ;
#21235=ORIENTED_EDGE('',*,*,#15882,.T.) ;
#21236=ORIENTED_EDGE('',*,*,#15891,.T.) ;
#21237=ORIENTED_EDGE('',*,*,#15896,.T.) ;
#21238=ORIENTED_EDGE('',*,*,#15894,.F.) ;
#21239=ORIENTED_EDGE('',*,*,#15897,.F.) ;
#21240=ORIENTED_EDGE('',*,*,#15898,.F.) ;
#21241=ORIENTED_EDGE('',*,*,#15899,.T.) ;
#21242=ORIENTED_EDGE('',*,*,#15892,.F.) ;
#21243=ORIENTED_EDGE('',*,*,#15900,.F.) ;
#21244=ORIENTED_EDGE('',*,*,#15901,.F.) ;
#21245=ORIENTED_EDGE('',*,*,#15898,.T.) ;
#21246=ORIENTED_EDGE('',*,*,#15902,.T.) ;
#21247=ORIENTED_EDGE('',*,*,#15903,.F.) ;
#21248=ORIENTED_EDGE('',*,*,#15904,.F.) ;
#21249=ORIENTED_EDGE('',*,*,#15905,.T.) ;
#21250=ORIENTED_EDGE('',*,*,#15800,.T.) ;
#21251=ORIENTED_EDGE('',*,*,#15812,.T.) ;
#21252=ORIENTED_EDGE('',*,*,#15880,.T.) ;
#21253=ORIENTED_EDGE('',*,*,#15884,.T.) ;
#21254=ORIENTED_EDGE('',*,*,#15887,.T.) ;
#21255=ORIENTED_EDGE('',*,*,#15890,.T.) ;
#21256=ORIENTED_EDGE('',*,*,#15906,.F.) ;
#21257=ORIENTED_EDGE('',*,*,#15907,.T.) ;
#21258=ORIENTED_EDGE('',*,*,#15908,.T.) ;
#21259=ORIENTED_EDGE('',*,*,#15909,.F.) ;
#21260=ORIENTED_EDGE('',*,*,#15910,.T.) ;
#21261=ORIENTED_EDGE('',*,*,#15911,.T.) ;
#21262=ORIENTED_EDGE('',*,*,#15912,.T.) ;
#21263=ORIENTED_EDGE('',*,*,#15913,.T.) ;
#21264=ORIENTED_EDGE('',*,*,#15914,.T.) ;
#21265=ORIENTED_EDGE('',*,*,#15915,.F.) ;
#21266=ORIENTED_EDGE('',*,*,#15916,.F.) ;
#21267=ORIENTED_EDGE('',*,*,#15917,.T.) ;
#21268=ORIENTED_EDGE('',*,*,#15918,.F.) ;
#21269=ORIENTED_EDGE('',*,*,#15919,.F.) ;
#21270=ORIENTED_EDGE('',*,*,#15914,.F.) ;
#21271=ORIENTED_EDGE('',*,*,#15920,.F.) ;
#21272=ORIENTED_EDGE('',*,*,#15921,.F.) ;
#21273=ORIENTED_EDGE('',*,*,#15922,.T.) ;
#21274=ORIENTED_EDGE('',*,*,#15907,.F.) ;
#21275=ORIENTED_EDGE('',*,*,#15923,.F.) ;
#21276=ORIENTED_EDGE('',*,*,#15924,.F.) ;
#21277=ORIENTED_EDGE('',*,*,#15925,.T.) ;
#21278=ORIENTED_EDGE('',*,*,#15912,.F.) ;
#21279=ORIENTED_EDGE('',*,*,#15926,.T.) ;
#21280=ORIENTED_EDGE('',*,*,#15927,.F.) ;
#21281=ORIENTED_EDGE('',*,*,#15928,.F.) ;
#21282=ORIENTED_EDGE('',*,*,#15929,.F.) ;
#21283=ORIENTED_EDGE('',*,*,#15920,.T.) ;
#21284=ORIENTED_EDGE('',*,*,#15913,.F.) ;
#21285=ORIENTED_EDGE('',*,*,#15925,.F.) ;
#21286=ORIENTED_EDGE('',*,*,#15930,.F.) ;
#21287=ORIENTED_EDGE('',*,*,#15931,.T.) ;
#21288=ORIENTED_EDGE('',*,*,#15932,.T.) ;
#21289=ORIENTED_EDGE('',*,*,#15933,.T.) ;
#21290=ORIENTED_EDGE('',*,*,#15934,.F.) ;
#21291=ORIENTED_EDGE('',*,*,#15909,.T.) ;
#21292=ORIENTED_EDGE('',*,*,#15935,.T.) ;
#21293=ORIENTED_EDGE('',*,*,#15936,.T.) ;
#21294=ORIENTED_EDGE('',*,*,#15937,.T.) ;
#21295=ORIENTED_EDGE('',*,*,#15933,.F.) ;
#21296=ORIENTED_EDGE('',*,*,#15938,.F.) ;
#21297=ORIENTED_EDGE('',*,*,#15939,.F.) ;
#21298=ORIENTED_EDGE('',*,*,#15940,.T.) ;
#21299=ORIENTED_EDGE('',*,*,#15941,.F.) ;
#21300=ORIENTED_EDGE('',*,*,#15942,.F.) ;
#21301=ORIENTED_EDGE('',*,*,#15943,.F.) ;
#21302=ORIENTED_EDGE('',*,*,#15944,.F.) ;
#21303=ORIENTED_EDGE('',*,*,#15945,.F.) ;
#21304=ORIENTED_EDGE('',*,*,#15946,.F.) ;
#21305=ORIENTED_EDGE('',*,*,#15947,.F.) ;
#21306=ORIENTED_EDGE('',*,*,#15948,.F.) ;
#21307=ORIENTED_EDGE('',*,*,#15949,.F.) ;
#21308=ORIENTED_EDGE('',*,*,#15950,.T.) ;
#21309=ORIENTED_EDGE('',*,*,#15951,.F.) ;
#21310=ORIENTED_EDGE('',*,*,#15952,.T.) ;
#21311=ORIENTED_EDGE('',*,*,#15936,.F.) ;
#21312=ORIENTED_EDGE('',*,*,#15953,.T.) ;
#21313=ORIENTED_EDGE('',*,*,#15954,.F.) ;
#21314=ORIENTED_EDGE('',*,*,#15955,.F.) ;
#21315=ORIENTED_EDGE('',*,*,#15956,.F.) ;
#21316=ORIENTED_EDGE('',*,*,#15957,.F.) ;
#21317=ORIENTED_EDGE('',*,*,#15958,.T.) ;
#21318=ORIENTED_EDGE('',*,*,#15959,.T.) ;
#21319=ORIENTED_EDGE('',*,*,#15960,.T.) ;
#21320=ORIENTED_EDGE('',*,*,#15961,.F.) ;
#21321=ORIENTED_EDGE('',*,*,#15962,.F.) ;
#21322=ORIENTED_EDGE('',*,*,#15963,.T.) ;
#21323=ORIENTED_EDGE('',*,*,#15964,.T.) ;
#21324=ORIENTED_EDGE('',*,*,#15965,.F.) ;
#21325=ORIENTED_EDGE('',*,*,#15966,.T.) ;
#21326=ORIENTED_EDGE('',*,*,#15967,.T.) ;
#21327=ORIENTED_EDGE('',*,*,#15968,.T.) ;
#21328=ORIENTED_EDGE('',*,*,#15969,.F.) ;
#21329=ORIENTED_EDGE('',*,*,#15956,.T.) ;
#21330=ORIENTED_EDGE('',*,*,#15962,.T.) ;
#21331=ORIENTED_EDGE('',*,*,#15970,.F.) ;
#21332=ORIENTED_EDGE('',*,*,#15971,.F.) ;
#21333=ORIENTED_EDGE('',*,*,#15952,.F.) ;
#21334=ORIENTED_EDGE('',*,*,#15972,.T.) ;
#21335=ORIENTED_EDGE('',*,*,#15973,.F.) ;
#21336=ORIENTED_EDGE('',*,*,#15974,.F.) ;
#21337=ORIENTED_EDGE('',*,*,#15975,.F.) ;
#21338=ORIENTED_EDGE('',*,*,#15976,.F.) ;
#21339=ORIENTED_EDGE('',*,*,#15977,.T.) ;
#21340=ORIENTED_EDGE('',*,*,#15978,.T.) ;
#21341=ORIENTED_EDGE('',*,*,#15979,.F.) ;
#21342=ORIENTED_EDGE('',*,*,#15980,.F.) ;
#21343=ORIENTED_EDGE('',*,*,#15981,.T.) ;
#21344=ORIENTED_EDGE('',*,*,#15871,.F.) ;
#21345=ORIENTED_EDGE('',*,*,#15982,.T.) ;
#21346=ORIENTED_EDGE('',*,*,#15983,.F.) ;
#21347=ORIENTED_EDGE('',*,*,#15984,.T.) ;
#21348=ORIENTED_EDGE('',*,*,#15953,.F.) ;
#21349=ORIENTED_EDGE('',*,*,#15935,.F.) ;
#21350=ORIENTED_EDGE('',*,*,#15908,.F.) ;
#21351=ORIENTED_EDGE('',*,*,#15922,.F.) ;
#21352=ORIENTED_EDGE('',*,*,#15985,.F.) ;
#21353=ORIENTED_EDGE('',*,*,#15986,.T.) ;
#21354=ORIENTED_EDGE('',*,*,#15987,.F.) ;
#21355=ORIENTED_EDGE('',*,*,#15988,.F.) ;
#21356=ORIENTED_EDGE('',*,*,#15975,.T.) ;
#21357=ORIENTED_EDGE('',*,*,#15949,.T.) ;
#21358=ORIENTED_EDGE('',*,*,#15971,.T.) ;
#21359=ORIENTED_EDGE('',*,*,#15989,.F.) ;
#21360=ORIENTED_EDGE('',*,*,#15990,.F.) ;
#21361=ORIENTED_EDGE('',*,*,#15951,.T.) ;
#21362=ORIENTED_EDGE('',*,*,#15991,.T.) ;
#21363=ORIENTED_EDGE('',*,*,#15992,.F.) ;
#21364=ORIENTED_EDGE('',*,*,#15972,.F.) ;
#21365=ORIENTED_EDGE('',*,*,#15948,.T.) ;
#21366=ORIENTED_EDGE('',*,*,#15993,.T.) ;
#21367=ORIENTED_EDGE('',*,*,#15994,.F.) ;
#21368=ORIENTED_EDGE('',*,*,#15995,.F.) ;
#21369=ORIENTED_EDGE('',*,*,#15945,.T.) ;
#21370=ORIENTED_EDGE('',*,*,#15995,.T.) ;
#21371=ORIENTED_EDGE('',*,*,#15996,.F.) ;
#21372=ORIENTED_EDGE('',*,*,#15997,.F.) ;
#21373=ORIENTED_EDGE('',*,*,#15944,.T.) ;
#21374=ORIENTED_EDGE('',*,*,#15998,.T.) ;
#21375=ORIENTED_EDGE('',*,*,#15999,.F.) ;
#21376=ORIENTED_EDGE('',*,*,#16000,.F.) ;
#21377=ORIENTED_EDGE('',*,*,#15941,.T.) ;
#21378=ORIENTED_EDGE('',*,*,#16000,.T.) ;
#21379=ORIENTED_EDGE('',*,*,#16001,.F.) ;
#21380=ORIENTED_EDGE('',*,*,#16002,.F.) ;
#21381=ORIENTED_EDGE('',*,*,#16003,.T.) ;
#21382=ORIENTED_EDGE('',*,*,#15989,.T.) ;
#21383=ORIENTED_EDGE('',*,*,#15970,.T.) ;
#21384=ORIENTED_EDGE('',*,*,#15961,.T.) ;
#21385=ORIENTED_EDGE('',*,*,#16004,.T.) ;
#21386=ORIENTED_EDGE('',*,*,#16005,.T.) ;
#21387=ORIENTED_EDGE('',*,*,#15996,.T.) ;
#21388=ORIENTED_EDGE('',*,*,#15994,.T.) ;
#21389=ORIENTED_EDGE('',*,*,#16006,.T.) ;
#21390=ORIENTED_EDGE('',*,*,#16007,.T.) ;
#21391=ORIENTED_EDGE('',*,*,#15957,.T.) ;
#21392=ORIENTED_EDGE('',*,*,#15969,.T.) ;
#21393=ORIENTED_EDGE('',*,*,#16008,.T.) ;
#21394=ORIENTED_EDGE('',*,*,#16009,.T.) ;
#21395=ORIENTED_EDGE('',*,*,#16010,.T.) ;
#21396=ORIENTED_EDGE('',*,*,#16011,.T.) ;
#21397=ORIENTED_EDGE('',*,*,#15973,.T.) ;
#21398=ORIENTED_EDGE('',*,*,#15992,.T.) ;
#21399=ORIENTED_EDGE('',*,*,#16012,.T.) ;
#21400=ORIENTED_EDGE('',*,*,#16013,.T.) ;
#21401=ORIENTED_EDGE('',*,*,#16001,.T.) ;
#21402=ORIENTED_EDGE('',*,*,#15999,.T.) ;
#21403=ORIENTED_EDGE('',*,*,#16014,.F.) ;
#21404=ORIENTED_EDGE('',*,*,#16015,.T.) ;
#21405=ORIENTED_EDGE('',*,*,#16016,.F.) ;
#21406=ORIENTED_EDGE('',*,*,#15980,.T.) ;
#21407=ORIENTED_EDGE('',*,*,#16017,.T.) ;
#21408=ORIENTED_EDGE('',*,*,#16018,.F.) ;
#21409=ORIENTED_EDGE('',*,*,#16014,.T.) ;
#21410=ORIENTED_EDGE('',*,*,#15979,.T.) ;
#21411=ORIENTED_EDGE('',*,*,#15974,.T.) ;
#21412=ORIENTED_EDGE('',*,*,#16011,.F.) ;
#21413=ORIENTED_EDGE('',*,*,#16019,.F.) ;
#21414=ORIENTED_EDGE('',*,*,#16020,.T.) ;
#21415=ORIENTED_EDGE('',*,*,#15947,.T.) ;
#21416=ORIENTED_EDGE('',*,*,#16021,.T.) ;
#21417=ORIENTED_EDGE('',*,*,#16004,.F.) ;
#21418=ORIENTED_EDGE('',*,*,#15993,.F.) ;
#21419=ORIENTED_EDGE('',*,*,#15946,.T.) ;
#21420=ORIENTED_EDGE('',*,*,#15997,.T.) ;
#21421=ORIENTED_EDGE('',*,*,#16005,.F.) ;
#21422=ORIENTED_EDGE('',*,*,#16021,.F.) ;
#21423=ORIENTED_EDGE('',*,*,#15943,.T.) ;
#21424=ORIENTED_EDGE('',*,*,#16022,.T.) ;
#21425=ORIENTED_EDGE('',*,*,#16012,.F.) ;
#21426=ORIENTED_EDGE('',*,*,#15998,.F.) ;
#21427=ORIENTED_EDGE('',*,*,#15942,.T.) ;
#21428=ORIENTED_EDGE('',*,*,#16002,.T.) ;
#21429=ORIENTED_EDGE('',*,*,#16013,.F.) ;
#21430=ORIENTED_EDGE('',*,*,#16022,.F.) ;
#21431=ORIENTED_EDGE('',*,*,#16023,.T.) ;
#21432=ORIENTED_EDGE('',*,*,#16024,.T.) ;
#21433=ORIENTED_EDGE('',*,*,#16025,.T.) ;
#21434=ORIENTED_EDGE('',*,*,#16026,.T.) ;
#21435=ORIENTED_EDGE('',*,*,#15986,.F.) ;
#21436=ORIENTED_EDGE('',*,*,#16027,.T.) ;
#21437=ORIENTED_EDGE('',*,*,#16025,.F.) ;
#21438=ORIENTED_EDGE('',*,*,#16027,.F.) ;
#21439=ORIENTED_EDGE('',*,*,#16020,.F.) ;
#21440=ORIENTED_EDGE('',*,*,#16023,.F.) ;
#21441=ORIENTED_EDGE('',*,*,#16028,.T.) ;
#21442=ORIENTED_EDGE('',*,*,#15959,.F.) ;
#21443=ORIENTED_EDGE('',*,*,#15963,.F.) ;
#21444=ORIENTED_EDGE('',*,*,#16028,.F.) ;
#21445=ORIENTED_EDGE('',*,*,#16026,.F.) ;
#21446=ORIENTED_EDGE('',*,*,#16029,.T.) ;
#21447=ORIENTED_EDGE('',*,*,#16009,.F.) ;
#21448=ORIENTED_EDGE('',*,*,#16029,.F.) ;
#21449=ORIENTED_EDGE('',*,*,#16008,.F.) ;
#21450=ORIENTED_EDGE('',*,*,#16030,.T.) ;
#21451=ORIENTED_EDGE('',*,*,#16024,.F.) ;
#21452=ORIENTED_EDGE('',*,*,#16030,.F.) ;
#21453=ORIENTED_EDGE('',*,*,#16031,.T.) ;
#21454=ORIENTED_EDGE('',*,*,#16032,.T.) ;
#21455=ORIENTED_EDGE('',*,*,#16033,.T.) ;
#21456=ORIENTED_EDGE('',*,*,#15965,.T.) ;
#21457=ORIENTED_EDGE('',*,*,#16034,.T.) ;
#21458=ORIENTED_EDGE('',*,*,#16035,.F.) ;
#21459=ORIENTED_EDGE('',*,*,#16036,.F.) ;
#21460=ORIENTED_EDGE('',*,*,#16037,.F.) ;
#21461=ORIENTED_EDGE('',*,*,#16038,.T.) ;
#21462=ORIENTED_EDGE('',*,*,#16039,.F.) ;
#21463=ORIENTED_EDGE('',*,*,#16040,.F.) ;
#21464=ORIENTED_EDGE('',*,*,#16041,.F.) ;
#21465=ORIENTED_EDGE('',*,*,#16037,.T.) ;
#21466=ORIENTED_EDGE('',*,*,#16042,.T.) ;
#21467=ORIENTED_EDGE('',*,*,#16041,.T.) ;
#21468=ORIENTED_EDGE('',*,*,#16043,.T.) ;
#21469=ORIENTED_EDGE('',*,*,#16044,.F.) ;
#21470=ORIENTED_EDGE('',*,*,#16045,.T.) ;
#21471=ORIENTED_EDGE('',*,*,#16035,.T.) ;
#21472=ORIENTED_EDGE('',*,*,#16046,.T.) ;
#21473=ORIENTED_EDGE('',*,*,#15967,.F.) ;
#21474=ORIENTED_EDGE('',*,*,#16047,.T.) ;
#21475=ORIENTED_EDGE('',*,*,#16039,.T.) ;
#21476=ORIENTED_EDGE('',*,*,#16048,.T.) ;
#21477=ORIENTED_EDGE('',*,*,#16049,.F.) ;
#21478=ORIENTED_EDGE('',*,*,#16046,.F.) ;
#21479=ORIENTED_EDGE('',*,*,#16034,.F.) ;
#21480=ORIENTED_EDGE('',*,*,#16043,.F.) ;
#21481=ORIENTED_EDGE('',*,*,#16040,.T.) ;
#21482=ORIENTED_EDGE('',*,*,#16047,.F.) ;
#21483=ORIENTED_EDGE('',*,*,#15966,.F.) ;
#21484=ORIENTED_EDGE('',*,*,#16033,.F.) ;
#21485=ORIENTED_EDGE('',*,*,#15860,.T.) ;
#21486=ORIENTED_EDGE('',*,*,#16050,.F.) ;
#21487=ORIENTED_EDGE('',*,*,#16006,.F.) ;
#21488=ORIENTED_EDGE('',*,*,#15968,.F.) ;
#21489=ORIENTED_EDGE('',*,*,#16048,.F.) ;
#21490=ORIENTED_EDGE('',*,*,#16038,.F.) ;
#21491=ORIENTED_EDGE('',*,*,#16042,.F.) ;
#21492=ORIENTED_EDGE('',*,*,#16036,.T.) ;
#21493=ORIENTED_EDGE('',*,*,#16045,.F.) ;
#21494=ORIENTED_EDGE('',*,*,#15862,.T.) ;
#21495=ORIENTED_EDGE('',*,*,#16051,.T.) ;
#21496=ORIENTED_EDGE('',*,*,#16052,.T.) ;
#21497=ORIENTED_EDGE('',*,*,#16053,.T.) ;
#21498=ORIENTED_EDGE('',*,*,#16054,.T.) ;
#21499=ORIENTED_EDGE('',*,*,#16055,.T.) ;
#21500=ORIENTED_EDGE('',*,*,#15916,.T.) ;
#21501=ORIENTED_EDGE('',*,*,#16056,.F.) ;
#21502=ORIENTED_EDGE('',*,*,#15931,.F.) ;
#21503=ORIENTED_EDGE('',*,*,#15929,.T.) ;
#21504=ORIENTED_EDGE('',*,*,#15806,.T.) ;
#21505=ORIENTED_EDGE('',*,*,#15836,.T.) ;
#21506=ORIENTED_EDGE('',*,*,#15919,.T.) ;
#21507=ORIENTED_EDGE('',*,*,#16057,.F.) ;
#21508=ORIENTED_EDGE('',*,*,#15926,.F.) ;
#21509=ORIENTED_EDGE('',*,*,#15911,.F.) ;
#21510=ORIENTED_EDGE('',*,*,#15928,.T.) ;
#21511=ORIENTED_EDGE('',*,*,#16058,.F.) ;
#21512=ORIENTED_EDGE('',*,*,#15917,.F.) ;
#21513=ORIENTED_EDGE('',*,*,#16055,.F.) ;
#21514=ORIENTED_EDGE('',*,*,#16057,.T.) ;
#21515=ORIENTED_EDGE('',*,*,#15918,.T.) ;
#21516=ORIENTED_EDGE('',*,*,#16058,.T.) ;
#21517=ORIENTED_EDGE('',*,*,#15927,.T.) ;
#21518=ORIENTED_EDGE('',*,*,#16059,.T.) ;
#21519=ORIENTED_EDGE('',*,*,#16060,.T.) ;
#21520=ORIENTED_EDGE('',*,*,#16061,.T.) ;
#21521=ORIENTED_EDGE('',*,*,#16062,.T.) ;
#21522=ORIENTED_EDGE('',*,*,#16054,.F.) ;
#21523=ORIENTED_EDGE('',*,*,#16063,.T.) ;
#21524=ORIENTED_EDGE('',*,*,#16062,.F.) ;
#21525=ORIENTED_EDGE('',*,*,#16064,.F.) ;
#21526=ORIENTED_EDGE('',*,*,#16053,.F.) ;
#21527=ORIENTED_EDGE('',*,*,#16065,.T.) ;
#21528=ORIENTED_EDGE('',*,*,#16059,.F.) ;
#21529=ORIENTED_EDGE('',*,*,#16063,.F.) ;
#21530=ORIENTED_EDGE('',*,*,#16052,.F.) ;
#21531=ORIENTED_EDGE('',*,*,#16066,.T.) ;
#21532=ORIENTED_EDGE('',*,*,#16060,.F.) ;
#21533=ORIENTED_EDGE('',*,*,#16065,.F.) ;
#21534=ORIENTED_EDGE('',*,*,#16051,.F.) ;
#21535=ORIENTED_EDGE('',*,*,#16064,.T.) ;
#21536=ORIENTED_EDGE('',*,*,#16061,.F.) ;
#21537=ORIENTED_EDGE('',*,*,#16066,.F.) ;
#21538=ORIENTED_EDGE('',*,*,#16067,.T.) ;
#21539=ORIENTED_EDGE('',*,*,#16068,.T.) ;
#21540=ORIENTED_EDGE('',*,*,#16069,.T.) ;
#21541=ORIENTED_EDGE('',*,*,#16068,.F.) ;
#21542=ORIENTED_EDGE('',*,*,#16070,.T.) ;
#21543=ORIENTED_EDGE('',*,*,#16071,.F.) ;
#21544=ORIENTED_EDGE('',*,*,#16070,.F.) ;
#21545=ORIENTED_EDGE('',*,*,#15910,.F.) ;
#21546=ORIENTED_EDGE('',*,*,#16072,.T.) ;
#21547=ORIENTED_EDGE('',*,*,#16069,.F.) ;
#21548=ORIENTED_EDGE('',*,*,#16072,.F.) ;
#21549=ORIENTED_EDGE('',*,*,#15930,.T.) ;
#21550=ORIENTED_EDGE('',*,*,#15924,.T.) ;
#21551=ORIENTED_EDGE('',*,*,#16017,.F.) ;
#21552=ORIENTED_EDGE('',*,*,#15985,.T.) ;
#21553=ORIENTED_EDGE('',*,*,#15921,.T.) ;
#21554=ORIENTED_EDGE('',*,*,#15805,.T.) ;
#21555=ORIENTED_EDGE('',*,*,#15835,.T.) ;
#21556=ORIENTED_EDGE('',*,*,#16071,.T.) ;
#21557=ORIENTED_EDGE('',*,*,#16073,.T.) ;
#21558=ORIENTED_EDGE('',*,*,#16074,.T.) ;
#21559=ORIENTED_EDGE('',*,*,#16075,.T.) ;
#21560=ORIENTED_EDGE('',*,*,#16074,.F.) ;
#21561=ORIENTED_EDGE('',*,*,#16076,.T.) ;
#21562=ORIENTED_EDGE('',*,*,#16073,.F.) ;
#21563=ORIENTED_EDGE('',*,*,#16076,.F.) ;
#21564=ORIENTED_EDGE('',*,*,#16067,.F.) ;
#21565=ORIENTED_EDGE('',*,*,#16077,.T.) ;
#21566=ORIENTED_EDGE('',*,*,#16075,.F.) ;
#21567=ORIENTED_EDGE('',*,*,#16077,.F.) ;
#21568=ORIENTED_EDGE('',*,*,#16078,.T.) ;
#21569=ORIENTED_EDGE('',*,*,#16079,.T.) ;
#21570=ORIENTED_EDGE('',*,*,#15904,.T.) ;
#21571=ORIENTED_EDGE('',*,*,#16080,.F.) ;
#21572=ORIENTED_EDGE('',*,*,#15938,.T.) ;
#21573=ORIENTED_EDGE('',*,*,#15932,.F.) ;
#21574=ORIENTED_EDGE('',*,*,#16056,.T.) ;
#21575=ORIENTED_EDGE('',*,*,#15915,.T.) ;
#21576=ORIENTED_EDGE('',*,*,#15906,.T.) ;
#21577=ORIENTED_EDGE('',*,*,#15937,.F.) ;
#21578=ORIENTED_EDGE('',*,*,#15955,.T.) ;
#21579=ORIENTED_EDGE('',*,*,#16081,.F.) ;
#21580=ORIENTED_EDGE('',*,*,#16082,.T.) ;
#21581=ORIENTED_EDGE('',*,*,#16081,.T.) ;
#21582=ORIENTED_EDGE('',*,*,#15954,.T.) ;
#21583=ORIENTED_EDGE('',*,*,#15984,.F.) ;
#21584=ORIENTED_EDGE('',*,*,#15872,.T.) ;
#21585=ORIENTED_EDGE('',*,*,#15981,.F.) ;
#21586=ORIENTED_EDGE('',*,*,#16016,.T.) ;
#21587=ORIENTED_EDGE('',*,*,#16083,.T.) ;
#21588=ORIENTED_EDGE('',*,*,#15903,.T.) ;
#21589=ORIENTED_EDGE('',*,*,#16084,.T.) ;
#21590=ORIENTED_EDGE('',*,*,#15939,.T.) ;
#21591=ORIENTED_EDGE('',*,*,#16080,.T.) ;
#21592=ORIENTED_EDGE('',*,*,#16085,.T.) ;
#21593=ORIENTED_EDGE('',*,*,#16086,.F.) ;
#21594=ORIENTED_EDGE('',*,*,#16087,.F.) ;
#21595=ORIENTED_EDGE('',*,*,#15869,.F.) ;
#21596=ORIENTED_EDGE('',*,*,#16079,.F.) ;
#21597=ORIENTED_EDGE('',*,*,#16088,.F.) ;
#21598=ORIENTED_EDGE('',*,*,#15982,.F.) ;
#21599=ORIENTED_EDGE('',*,*,#15870,.F.) ;
#21600=ORIENTED_EDGE('',*,*,#16087,.T.) ;
#21601=ORIENTED_EDGE('',*,*,#16089,.F.) ;
#21602=ORIENTED_EDGE('',*,*,#15900,.T.) ;
#21603=ORIENTED_EDGE('',*,*,#15895,.F.) ;
#21604=ORIENTED_EDGE('',*,*,#15896,.F.) ;
#21605=ORIENTED_EDGE('',*,*,#15905,.F.) ;
#21606=ORIENTED_EDGE('',*,*,#15875,.T.) ;
#21607=ORIENTED_EDGE('',*,*,#16078,.F.) ;
#21608=ORIENTED_EDGE('',*,*,#16082,.F.) ;
#21609=ORIENTED_EDGE('',*,*,#15983,.T.) ;
#21610=ORIENTED_EDGE('',*,*,#16088,.T.) ;
#21611=ORIENTED_EDGE('',*,*,#15901,.T.) ;
#21612=ORIENTED_EDGE('',*,*,#16089,.T.) ;
#21613=ORIENTED_EDGE('',*,*,#16086,.T.) ;
#21614=ORIENTED_EDGE('',*,*,#16090,.T.) ;
#21615=ORIENTED_EDGE('',*,*,#16091,.T.) ;
#21616=ORIENTED_EDGE('',*,*,#15902,.F.) ;
#21617=ORIENTED_EDGE('',*,*,#15897,.T.) ;
#21618=ORIENTED_EDGE('',*,*,#15893,.F.) ;
#21619=ORIENTED_EDGE('',*,*,#15899,.F.) ;
#21620=ORIENTED_EDGE('',*,*,#16090,.F.) ;
#21621=ORIENTED_EDGE('',*,*,#16085,.F.) ;
#21622=ORIENTED_EDGE('',*,*,#15873,.F.) ;
#21623=ORIENTED_EDGE('',*,*,#16092,.T.) ;
#21624=ORIENTED_EDGE('',*,*,#15976,.T.) ;
#21625=ORIENTED_EDGE('',*,*,#15988,.T.) ;
#21626=ORIENTED_EDGE('',*,*,#16093,.T.) ;
#21627=ORIENTED_EDGE('',*,*,#16094,.T.) ;
#21628=ORIENTED_EDGE('',*,*,#16095,.T.) ;
#21629=ORIENTED_EDGE('',*,*,#16096,.T.) ;
#21630=ORIENTED_EDGE('',*,*,#16093,.F.) ;
#21631=ORIENTED_EDGE('',*,*,#15987,.T.) ;
#21632=ORIENTED_EDGE('',*,*,#16019,.T.) ;
#21633=ORIENTED_EDGE('',*,*,#16010,.F.) ;
#21634=ORIENTED_EDGE('',*,*,#15991,.F.) ;
#21635=ORIENTED_EDGE('',*,*,#15950,.F.) ;
#21636=ORIENTED_EDGE('',*,*,#15990,.T.) ;
#21637=ORIENTED_EDGE('',*,*,#16003,.F.) ;
#21638=ORIENTED_EDGE('',*,*,#15960,.F.) ;
#21639=ORIENTED_EDGE('',*,*,#15958,.F.) ;
#21640=ORIENTED_EDGE('',*,*,#16007,.F.) ;
#21641=ORIENTED_EDGE('',*,*,#16050,.T.) ;
#21642=ORIENTED_EDGE('',*,*,#16044,.T.) ;
#21643=ORIENTED_EDGE('',*,*,#16049,.T.) ;
#21644=ORIENTED_EDGE('',*,*,#16032,.F.) ;
#21645=ORIENTED_EDGE('',*,*,#15940,.F.) ;
#21646=ORIENTED_EDGE('',*,*,#16084,.F.) ;
#21647=ORIENTED_EDGE('',*,*,#16091,.F.) ;
#21648=ORIENTED_EDGE('',*,*,#16083,.F.) ;
#21649=ORIENTED_EDGE('',*,*,#16015,.F.) ;
#21650=ORIENTED_EDGE('',*,*,#16018,.T.) ;
#21651=ORIENTED_EDGE('',*,*,#15923,.T.) ;
#21652=ORIENTED_EDGE('',*,*,#15934,.T.) ;
#21653=ORIENTED_EDGE('',*,*,#16097,.T.) ;
#21654=ORIENTED_EDGE('',*,*,#16098,.F.) ;
#21655=ORIENTED_EDGE('',*,*,#16099,.F.) ;
#21656=ORIENTED_EDGE('',*,*,#16100,.F.) ;
#21657=ORIENTED_EDGE('',*,*,#16101,.T.) ;
#21658=ORIENTED_EDGE('',*,*,#16102,.F.) ;
#21659=ORIENTED_EDGE('',*,*,#16103,.F.) ;
#21660=ORIENTED_EDGE('',*,*,#16104,.F.) ;
#21661=ORIENTED_EDGE('',*,*,#16096,.F.) ;
#21662=ORIENTED_EDGE('',*,*,#16105,.F.) ;
#21663=ORIENTED_EDGE('',*,*,#16097,.F.) ;
#21664=ORIENTED_EDGE('',*,*,#16106,.F.) ;
#21665=ORIENTED_EDGE('',*,*,#16103,.T.) ;
#21666=ORIENTED_EDGE('',*,*,#16107,.F.) ;
#21667=ORIENTED_EDGE('',*,*,#15977,.F.) ;
#21668=ORIENTED_EDGE('',*,*,#16092,.F.) ;
#21669=ORIENTED_EDGE('',*,*,#15857,.T.) ;
#21670=ORIENTED_EDGE('',*,*,#16095,.F.) ;
#21671=ORIENTED_EDGE('',*,*,#16108,.T.) ;
#21672=ORIENTED_EDGE('',*,*,#16098,.T.) ;
#21673=ORIENTED_EDGE('',*,*,#16105,.T.) ;
#21674=ORIENTED_EDGE('',*,*,#16100,.T.) ;
#21675=ORIENTED_EDGE('',*,*,#16109,.T.) ;
#21676=ORIENTED_EDGE('',*,*,#16104,.T.) ;
#21677=ORIENTED_EDGE('',*,*,#16106,.T.) ;
#21678=ORIENTED_EDGE('',*,*,#16094,.F.) ;
#21679=ORIENTED_EDGE('',*,*,#16031,.F.) ;
#21680=ORIENTED_EDGE('',*,*,#15964,.F.) ;
#21681=ORIENTED_EDGE('',*,*,#16110,.F.) ;
#21682=ORIENTED_EDGE('',*,*,#16101,.F.) ;
#21683=ORIENTED_EDGE('',*,*,#16109,.F.) ;
#21684=ORIENTED_EDGE('',*,*,#16099,.T.) ;
#21685=ORIENTED_EDGE('',*,*,#16108,.F.) ;
#21686=ORIENTED_EDGE('',*,*,#15859,.T.) ;
#21687=ORIENTED_EDGE('',*,*,#15978,.F.) ;
#21688=ORIENTED_EDGE('',*,*,#16107,.T.) ;
#21689=ORIENTED_EDGE('',*,*,#16102,.T.) ;
#21690=ORIENTED_EDGE('',*,*,#16110,.T.) ;
#21691=ORIENTED_EDGE('',*,*,#16111,.F.) ;
#21692=ORIENTED_EDGE('',*,*,#16112,.F.) ;
#21693=ORIENTED_EDGE('',*,*,#16113,.F.) ;
#21694=ORIENTED_EDGE('',*,*,#16114,.F.) ;
#21695=ORIENTED_EDGE('',*,*,#16114,.T.) ;
#21696=ORIENTED_EDGE('',*,*,#16115,.F.) ;
#21697=ORIENTED_EDGE('',*,*,#16116,.T.) ;
#21698=ORIENTED_EDGE('',*,*,#16117,.T.) ;
#21699=ORIENTED_EDGE('',*,*,#16113,.T.) ;
#21700=ORIENTED_EDGE('',*,*,#16118,.F.) ;
#21701=ORIENTED_EDGE('',*,*,#16119,.T.) ;
#21702=ORIENTED_EDGE('',*,*,#16115,.T.) ;
#21703=ORIENTED_EDGE('',*,*,#16112,.T.) ;
#21704=ORIENTED_EDGE('',*,*,#16120,.F.) ;
#21705=ORIENTED_EDGE('',*,*,#16121,.T.) ;
#21706=ORIENTED_EDGE('',*,*,#16118,.T.) ;
#21707=ORIENTED_EDGE('',*,*,#16111,.T.) ;
#21708=ORIENTED_EDGE('',*,*,#16117,.F.) ;
#21709=ORIENTED_EDGE('',*,*,#16122,.T.) ;
#21710=ORIENTED_EDGE('',*,*,#16120,.T.) ;
#21711=ORIENTED_EDGE('',*,*,#16119,.F.) ;
#21712=ORIENTED_EDGE('',*,*,#16121,.F.) ;
#21713=ORIENTED_EDGE('',*,*,#16122,.F.) ;
#21714=ORIENTED_EDGE('',*,*,#16116,.F.) ;
#21715=ORIENTED_EDGE('',*,*,#16123,.F.) ;
#21716=ORIENTED_EDGE('',*,*,#16124,.F.) ;
#21717=ORIENTED_EDGE('',*,*,#16125,.F.) ;
#21718=ORIENTED_EDGE('',*,*,#16126,.F.) ;
#21719=ORIENTED_EDGE('',*,*,#16127,.T.) ;
#21720=ORIENTED_EDGE('',*,*,#16128,.F.) ;
#21721=ORIENTED_EDGE('',*,*,#16125,.T.) ;
#21722=ORIENTED_EDGE('',*,*,#16129,.T.) ;
#21723=ORIENTED_EDGE('',*,*,#16130,.T.) ;
#21724=ORIENTED_EDGE('',*,*,#16129,.F.) ;
#21725=ORIENTED_EDGE('',*,*,#16124,.T.) ;
#21726=ORIENTED_EDGE('',*,*,#16131,.T.) ;
#21727=ORIENTED_EDGE('',*,*,#16132,.T.) ;
#21728=ORIENTED_EDGE('',*,*,#16131,.F.) ;
#21729=ORIENTED_EDGE('',*,*,#16123,.T.) ;
#21730=ORIENTED_EDGE('',*,*,#16133,.T.) ;
#21731=ORIENTED_EDGE('',*,*,#16134,.T.) ;
#21732=ORIENTED_EDGE('',*,*,#16133,.F.) ;
#21733=ORIENTED_EDGE('',*,*,#16126,.T.) ;
#21734=ORIENTED_EDGE('',*,*,#16128,.T.) ;
#21735=ORIENTED_EDGE('',*,*,#16127,.F.) ;
#21736=ORIENTED_EDGE('',*,*,#16130,.F.) ;
#21737=ORIENTED_EDGE('',*,*,#16132,.F.) ;
#21738=ORIENTED_EDGE('',*,*,#16134,.F.) ;
#21739=ORIENTED_EDGE('',*,*,#16135,.F.) ;
#21740=ORIENTED_EDGE('',*,*,#16136,.T.) ;
#21741=ORIENTED_EDGE('',*,*,#16137,.F.) ;
#21742=ORIENTED_EDGE('',*,*,#16138,.T.) ;
#21743=ORIENTED_EDGE('',*,*,#16139,.F.) ;
#21744=ORIENTED_EDGE('',*,*,#16136,.F.) ;
#21745=ORIENTED_EDGE('',*,*,#16140,.F.) ;
#21746=ORIENTED_EDGE('',*,*,#16138,.F.) ;
#21747=ORIENTED_EDGE('',*,*,#16140,.T.) ;
#21748=ORIENTED_EDGE('',*,*,#16135,.T.) ;
#21749=ORIENTED_EDGE('',*,*,#16139,.T.) ;
#21750=ORIENTED_EDGE('',*,*,#16137,.T.) ;
#21751=ORIENTED_EDGE('',*,*,#16141,.F.) ;
#21752=ORIENTED_EDGE('',*,*,#16142,.F.) ;
#21753=ORIENTED_EDGE('',*,*,#16143,.F.) ;
#21754=ORIENTED_EDGE('',*,*,#16144,.F.) ;
#21755=ORIENTED_EDGE('',*,*,#16145,.F.) ;
#21756=ORIENTED_EDGE('',*,*,#16144,.T.) ;
#21757=ORIENTED_EDGE('',*,*,#16146,.F.) ;
#21758=ORIENTED_EDGE('',*,*,#16147,.F.) ;
#21759=ORIENTED_EDGE('',*,*,#16145,.T.) ;
#21760=ORIENTED_EDGE('',*,*,#16148,.T.) ;
#21761=ORIENTED_EDGE('',*,*,#16141,.T.) ;
#21762=ORIENTED_EDGE('',*,*,#16146,.T.) ;
#21763=ORIENTED_EDGE('',*,*,#16143,.T.) ;
#21764=ORIENTED_EDGE('',*,*,#16149,.T.) ;
#21765=ORIENTED_EDGE('',*,*,#16147,.T.) ;
#21766=ORIENTED_EDGE('',*,*,#16149,.F.) ;
#21767=ORIENTED_EDGE('',*,*,#16142,.T.) ;
#21768=ORIENTED_EDGE('',*,*,#16148,.F.) ;
#21769=ORIENTED_EDGE('',*,*,#16150,.T.) ;
#21770=ORIENTED_EDGE('',*,*,#16151,.T.) ;
#21771=ORIENTED_EDGE('',*,*,#16152,.T.) ;
#21772=ORIENTED_EDGE('',*,*,#16153,.T.) ;
#21773=ORIENTED_EDGE('',*,*,#16152,.F.) ;
#21774=ORIENTED_EDGE('',*,*,#16154,.T.) ;
#21775=ORIENTED_EDGE('',*,*,#16155,.T.) ;
#21776=ORIENTED_EDGE('',*,*,#16156,.T.) ;
#21777=ORIENTED_EDGE('',*,*,#16155,.F.) ;
#21778=ORIENTED_EDGE('',*,*,#16157,.T.) ;
#21779=ORIENTED_EDGE('',*,*,#16158,.T.) ;
#21780=ORIENTED_EDGE('',*,*,#16157,.F.) ;
#21781=ORIENTED_EDGE('',*,*,#16154,.F.) ;
#21782=ORIENTED_EDGE('',*,*,#16151,.F.) ;
#21783=ORIENTED_EDGE('',*,*,#16156,.F.) ;
#21784=ORIENTED_EDGE('',*,*,#16158,.F.) ;
#21785=ORIENTED_EDGE('',*,*,#16150,.F.) ;
#21786=ORIENTED_EDGE('',*,*,#16153,.F.) ;
#21787=ORIENTED_EDGE('',*,*,#16159,.F.) ;
#21788=ORIENTED_EDGE('',*,*,#16160,.F.) ;
#21789=ORIENTED_EDGE('',*,*,#16161,.F.) ;
#21790=ORIENTED_EDGE('',*,*,#16162,.F.) ;
#21791=ORIENTED_EDGE('',*,*,#16163,.F.) ;
#21792=ORIENTED_EDGE('',*,*,#16164,.F.) ;
#21793=ORIENTED_EDGE('',*,*,#16165,.F.) ;
#21794=ORIENTED_EDGE('',*,*,#16160,.T.) ;
#21795=ORIENTED_EDGE('',*,*,#16163,.T.) ;
#21796=ORIENTED_EDGE('',*,*,#16159,.T.) ;
#21797=ORIENTED_EDGE('',*,*,#16166,.T.) ;
#21798=ORIENTED_EDGE('',*,*,#16165,.T.) ;
#21799=ORIENTED_EDGE('',*,*,#16167,.T.) ;
#21800=ORIENTED_EDGE('',*,*,#16161,.T.) ;
#21801=ORIENTED_EDGE('',*,*,#16164,.T.) ;
#21802=ORIENTED_EDGE('',*,*,#16166,.F.) ;
#21803=ORIENTED_EDGE('',*,*,#16162,.T.) ;
#21804=ORIENTED_EDGE('',*,*,#16167,.F.) ;
#21805=ORIENTED_EDGE('',*,*,#16168,.T.) ;
#21806=ORIENTED_EDGE('',*,*,#16169,.F.) ;
#21807=ORIENTED_EDGE('',*,*,#16170,.T.) ;
#21808=ORIENTED_EDGE('',*,*,#16171,.T.) ;
#21809=ORIENTED_EDGE('',*,*,#16172,.T.) ;
#21810=ORIENTED_EDGE('',*,*,#16173,.T.) ;
#21811=ORIENTED_EDGE('',*,*,#16174,.T.) ;
#21812=ORIENTED_EDGE('',*,*,#16170,.F.) ;
#21813=ORIENTED_EDGE('',*,*,#16175,.F.) ;
#21814=ORIENTED_EDGE('',*,*,#16172,.F.) ;
#21815=ORIENTED_EDGE('',*,*,#16176,.T.) ;
#21816=ORIENTED_EDGE('',*,*,#16173,.F.) ;
#21817=ORIENTED_EDGE('',*,*,#16175,.T.) ;
#21818=ORIENTED_EDGE('',*,*,#16169,.T.) ;
#21819=ORIENTED_EDGE('',*,*,#16168,.F.) ;
#21820=ORIENTED_EDGE('',*,*,#16174,.F.) ;
#21821=ORIENTED_EDGE('',*,*,#16171,.F.) ;
#21822=ORIENTED_EDGE('',*,*,#16176,.F.) ;
#21823=ORIENTED_EDGE('',*,*,#16177,.F.) ;
#21824=ORIENTED_EDGE('',*,*,#16178,.F.) ;
#21825=ORIENTED_EDGE('',*,*,#16179,.F.) ;
#21826=ORIENTED_EDGE('',*,*,#16180,.F.) ;
#21827=ORIENTED_EDGE('',*,*,#16178,.T.) ;
#21828=ORIENTED_EDGE('',*,*,#16181,.F.) ;
#21829=ORIENTED_EDGE('',*,*,#16182,.F.) ;
#21830=ORIENTED_EDGE('',*,*,#16183,.F.) ;
#21831=ORIENTED_EDGE('',*,*,#16177,.T.) ;
#21832=ORIENTED_EDGE('',*,*,#16184,.F.) ;
#21833=ORIENTED_EDGE('',*,*,#16181,.T.) ;
#21834=ORIENTED_EDGE('',*,*,#16180,.T.) ;
#21835=ORIENTED_EDGE('',*,*,#16185,.F.) ;
#21836=ORIENTED_EDGE('',*,*,#16182,.T.) ;
#21837=ORIENTED_EDGE('',*,*,#16184,.T.) ;
#21838=ORIENTED_EDGE('',*,*,#16179,.T.) ;
#21839=ORIENTED_EDGE('',*,*,#16183,.T.) ;
#21840=ORIENTED_EDGE('',*,*,#16185,.T.) ;
#21841=ORIENTED_EDGE('',*,*,#16186,.T.) ;
#21842=ORIENTED_EDGE('',*,*,#16187,.F.) ;
#21843=ORIENTED_EDGE('',*,*,#16188,.T.) ;
#21844=ORIENTED_EDGE('',*,*,#16189,.T.) ;
#21845=ORIENTED_EDGE('',*,*,#16190,.T.) ;
#21846=ORIENTED_EDGE('',*,*,#16191,.T.) ;
#21847=ORIENTED_EDGE('',*,*,#16192,.T.) ;
#21848=ORIENTED_EDGE('',*,*,#16188,.F.) ;
#21849=ORIENTED_EDGE('',*,*,#16193,.F.) ;
#21850=ORIENTED_EDGE('',*,*,#16190,.F.) ;
#21851=ORIENTED_EDGE('',*,*,#16194,.T.) ;
#21852=ORIENTED_EDGE('',*,*,#16191,.F.) ;
#21853=ORIENTED_EDGE('',*,*,#16193,.T.) ;
#21854=ORIENTED_EDGE('',*,*,#16187,.T.) ;
#21855=ORIENTED_EDGE('',*,*,#16186,.F.) ;
#21856=ORIENTED_EDGE('',*,*,#16192,.F.) ;
#21857=ORIENTED_EDGE('',*,*,#16189,.F.) ;
#21858=ORIENTED_EDGE('',*,*,#16194,.F.) ;
#21859=ORIENTED_EDGE('',*,*,#16195,.F.) ;
#21860=ORIENTED_EDGE('',*,*,#16196,.F.) ;
#21861=ORIENTED_EDGE('',*,*,#16197,.F.) ;
#21862=ORIENTED_EDGE('',*,*,#16198,.F.) ;
#21863=ORIENTED_EDGE('',*,*,#16198,.T.) ;
#21864=ORIENTED_EDGE('',*,*,#16199,.T.) ;
#21865=ORIENTED_EDGE('',*,*,#16196,.T.) ;
#21866=ORIENTED_EDGE('',*,*,#16200,.T.) ;
#21867=ORIENTED_EDGE('',*,*,#16197,.T.) ;
#21868=ORIENTED_EDGE('',*,*,#16200,.F.) ;
#21869=ORIENTED_EDGE('',*,*,#16195,.T.) ;
#21870=ORIENTED_EDGE('',*,*,#16199,.F.) ;
#21871=ORIENTED_EDGE('',*,*,#16201,.T.) ;
#21872=ORIENTED_EDGE('',*,*,#16202,.F.) ;
#21873=ORIENTED_EDGE('',*,*,#16203,.T.) ;
#21874=ORIENTED_EDGE('',*,*,#16204,.F.) ;
#21875=ORIENTED_EDGE('',*,*,#16205,.T.) ;
#21876=ORIENTED_EDGE('',*,*,#16204,.T.) ;
#21877=ORIENTED_EDGE('',*,*,#16206,.T.) ;
#21878=ORIENTED_EDGE('',*,*,#16202,.T.) ;
#21879=ORIENTED_EDGE('',*,*,#16205,.F.) ;
#21880=ORIENTED_EDGE('',*,*,#16203,.F.) ;
#21881=ORIENTED_EDGE('',*,*,#16206,.F.) ;
#21882=ORIENTED_EDGE('',*,*,#16201,.F.) ;
#21883=ORIENTED_EDGE('',*,*,#16207,.F.) ;
#21884=ORIENTED_EDGE('',*,*,#16208,.F.) ;
#21885=ORIENTED_EDGE('',*,*,#16209,.F.) ;
#21886=ORIENTED_EDGE('',*,*,#16210,.F.) ;
#21887=ORIENTED_EDGE('',*,*,#16209,.T.) ;
#21888=ORIENTED_EDGE('',*,*,#16211,.T.) ;
#21889=ORIENTED_EDGE('',*,*,#16207,.T.) ;
#21890=ORIENTED_EDGE('',*,*,#16212,.T.) ;
#21891=ORIENTED_EDGE('',*,*,#16210,.T.) ;
#21892=ORIENTED_EDGE('',*,*,#16211,.F.) ;
#21893=ORIENTED_EDGE('',*,*,#16208,.T.) ;
#21894=ORIENTED_EDGE('',*,*,#16212,.F.) ;
#21895=ORIENTED_EDGE('',*,*,#16213,.T.) ;
#21896=ORIENTED_EDGE('',*,*,#16214,.F.) ;
#21897=ORIENTED_EDGE('',*,*,#16215,.T.) ;
#21898=ORIENTED_EDGE('',*,*,#16216,.F.) ;
#21899=ORIENTED_EDGE('',*,*,#16217,.T.) ;
#21900=ORIENTED_EDGE('',*,*,#16214,.T.) ;
#21901=ORIENTED_EDGE('',*,*,#16218,.T.) ;
#21902=ORIENTED_EDGE('',*,*,#16216,.T.) ;
#21903=ORIENTED_EDGE('',*,*,#16215,.F.) ;
#21904=ORIENTED_EDGE('',*,*,#16217,.F.) ;
#21905=ORIENTED_EDGE('',*,*,#16213,.F.) ;
#21906=ORIENTED_EDGE('',*,*,#16218,.F.) ;
#21907=ORIENTED_EDGE('',*,*,#16219,.F.) ;
#21908=ORIENTED_EDGE('',*,*,#16220,.F.) ;
#21909=ORIENTED_EDGE('',*,*,#16221,.F.) ;
#21910=ORIENTED_EDGE('',*,*,#16222,.F.) ;
#21911=ORIENTED_EDGE('',*,*,#16220,.T.) ;
#21912=ORIENTED_EDGE('',*,*,#16223,.T.) ;
#21913=ORIENTED_EDGE('',*,*,#16221,.T.) ;
#21914=ORIENTED_EDGE('',*,*,#16223,.F.) ;
#21915=ORIENTED_EDGE('',*,*,#16219,.T.) ;
#21916=ORIENTED_EDGE('',*,*,#16224,.F.) ;
#21917=ORIENTED_EDGE('',*,*,#16222,.T.) ;
#21918=ORIENTED_EDGE('',*,*,#16224,.T.) ;
#21919=ORIENTED_EDGE('',*,*,#16225,.T.) ;
#21920=ORIENTED_EDGE('',*,*,#16226,.T.) ;
#21921=ORIENTED_EDGE('',*,*,#16227,.T.) ;
#21922=ORIENTED_EDGE('',*,*,#16228,.F.) ;
#21923=ORIENTED_EDGE('',*,*,#16229,.T.) ;
#21924=ORIENTED_EDGE('',*,*,#16230,.T.) ;
#21925=ORIENTED_EDGE('',*,*,#16231,.T.) ;
#21926=ORIENTED_EDGE('',*,*,#16226,.F.) ;
#21927=ORIENTED_EDGE('',*,*,#16232,.T.) ;
#21928=ORIENTED_EDGE('',*,*,#16228,.T.) ;
#21929=ORIENTED_EDGE('',*,*,#16233,.T.) ;
#21930=ORIENTED_EDGE('',*,*,#16234,.F.) ;
#21931=ORIENTED_EDGE('',*,*,#16235,.T.) ;
#21932=ORIENTED_EDGE('',*,*,#16234,.T.) ;
#21933=ORIENTED_EDGE('',*,*,#16236,.T.) ;
#21934=ORIENTED_EDGE('',*,*,#16230,.F.) ;
#21935=ORIENTED_EDGE('',*,*,#16236,.F.) ;
#21936=ORIENTED_EDGE('',*,*,#16233,.F.) ;
#21937=ORIENTED_EDGE('',*,*,#16227,.F.) ;
#21938=ORIENTED_EDGE('',*,*,#16231,.F.) ;
#21939=ORIENTED_EDGE('',*,*,#16235,.F.) ;
#21940=ORIENTED_EDGE('',*,*,#16229,.F.) ;
#21941=ORIENTED_EDGE('',*,*,#16225,.F.) ;
#21942=ORIENTED_EDGE('',*,*,#16232,.F.) ;
#21943=ORIENTED_EDGE('',*,*,#16237,.F.) ;
#21944=ORIENTED_EDGE('',*,*,#16238,.F.) ;
#21945=ORIENTED_EDGE('',*,*,#16239,.F.) ;
#21946=ORIENTED_EDGE('',*,*,#16240,.F.) ;
#21947=ORIENTED_EDGE('',*,*,#16241,.F.) ;
#21948=ORIENTED_EDGE('',*,*,#16242,.F.) ;
#21949=ORIENTED_EDGE('',*,*,#16243,.F.) ;
#21950=ORIENTED_EDGE('',*,*,#16244,.F.) ;
#21951=ORIENTED_EDGE('',*,*,#16237,.T.) ;
#21952=ORIENTED_EDGE('',*,*,#16245,.T.) ;
#21953=ORIENTED_EDGE('',*,*,#16241,.T.) ;
#21954=ORIENTED_EDGE('',*,*,#16246,.F.) ;
#21955=ORIENTED_EDGE('',*,*,#16240,.T.) ;
#21956=ORIENTED_EDGE('',*,*,#16247,.T.) ;
#21957=ORIENTED_EDGE('',*,*,#16242,.T.) ;
#21958=ORIENTED_EDGE('',*,*,#16245,.F.) ;
#21959=ORIENTED_EDGE('',*,*,#16238,.T.) ;
#21960=ORIENTED_EDGE('',*,*,#16246,.T.) ;
#21961=ORIENTED_EDGE('',*,*,#16244,.T.) ;
#21962=ORIENTED_EDGE('',*,*,#16248,.F.) ;
#21963=ORIENTED_EDGE('',*,*,#16239,.T.) ;
#21964=ORIENTED_EDGE('',*,*,#16248,.T.) ;
#21965=ORIENTED_EDGE('',*,*,#16243,.T.) ;
#21966=ORIENTED_EDGE('',*,*,#16247,.F.) ;
#21967=ORIENTED_EDGE('',*,*,#16249,.F.) ;
#21968=ORIENTED_EDGE('',*,*,#16250,.F.) ;
#21969=ORIENTED_EDGE('',*,*,#16251,.F.) ;
#21970=ORIENTED_EDGE('',*,*,#16252,.F.) ;
#21971=ORIENTED_EDGE('',*,*,#16253,.F.) ;
#21972=ORIENTED_EDGE('',*,*,#16254,.T.) ;
#21973=ORIENTED_EDGE('',*,*,#16255,.F.) ;
#21974=ORIENTED_EDGE('',*,*,#16250,.T.) ;
#21975=ORIENTED_EDGE('',*,*,#16256,.F.) ;
#21976=ORIENTED_EDGE('',*,*,#16257,.F.) ;
#21977=ORIENTED_EDGE('',*,*,#16258,.F.) ;
#21978=ORIENTED_EDGE('',*,*,#16254,.F.) ;
#21979=ORIENTED_EDGE('',*,*,#16251,.T.) ;
#21980=ORIENTED_EDGE('',*,*,#16255,.T.) ;
#21981=ORIENTED_EDGE('',*,*,#16258,.T.) ;
#21982=ORIENTED_EDGE('',*,*,#16259,.T.) ;
#21983=ORIENTED_EDGE('',*,*,#16260,.T.) ;
#21984=ORIENTED_EDGE('',*,*,#16261,.T.) ;
#21985=ORIENTED_EDGE('',*,*,#16262,.T.) ;
#21986=ORIENTED_EDGE('',*,*,#16263,.T.) ;
#21987=ORIENTED_EDGE('',*,*,#16264,.F.) ;
#21988=ORIENTED_EDGE('',*,*,#16265,.T.) ;
#21989=ORIENTED_EDGE('',*,*,#16266,.F.) ;
#21990=ORIENTED_EDGE('',*,*,#16267,.T.) ;
#21991=ORIENTED_EDGE('',*,*,#16257,.T.) ;
#21992=ORIENTED_EDGE('',*,*,#16268,.F.) ;
#21993=ORIENTED_EDGE('',*,*,#16269,.T.) ;
#21994=ORIENTED_EDGE('',*,*,#16259,.F.) ;
#21995=ORIENTED_EDGE('',*,*,#16252,.T.) ;
#21996=ORIENTED_EDGE('',*,*,#16267,.F.) ;
#21997=ORIENTED_EDGE('',*,*,#16270,.F.) ;
#21998=ORIENTED_EDGE('',*,*,#16271,.F.) ;
#21999=ORIENTED_EDGE('',*,*,#16249,.T.) ;
#22000=ORIENTED_EDGE('',*,*,#16271,.T.) ;
#22001=ORIENTED_EDGE('',*,*,#16272,.F.) ;
#22002=ORIENTED_EDGE('',*,*,#16273,.T.) ;
#22003=ORIENTED_EDGE('',*,*,#16274,.F.) ;
#22004=ORIENTED_EDGE('',*,*,#16275,.T.) ;
#22005=ORIENTED_EDGE('',*,*,#16276,.T.) ;
#22006=ORIENTED_EDGE('',*,*,#16277,.T.) ;
#22007=ORIENTED_EDGE('',*,*,#16278,.T.) ;
#22008=ORIENTED_EDGE('',*,*,#16268,.T.) ;
#22009=ORIENTED_EDGE('',*,*,#16256,.T.) ;
#22010=ORIENTED_EDGE('',*,*,#16253,.T.) ;
#22011=ORIENTED_EDGE('',*,*,#16279,.F.) ;
#22012=ORIENTED_EDGE('',*,*,#16273,.F.) ;
#22013=ORIENTED_EDGE('',*,*,#16280,.F.) ;
#22014=ORIENTED_EDGE('',*,*,#16265,.F.) ;
#22015=ORIENTED_EDGE('',*,*,#16280,.T.) ;
#22016=ORIENTED_EDGE('',*,*,#16272,.T.) ;
#22017=ORIENTED_EDGE('',*,*,#16270,.T.) ;
#22018=ORIENTED_EDGE('',*,*,#16266,.T.) ;
#22019=ORIENTED_EDGE('',*,*,#16279,.T.) ;
#22020=ORIENTED_EDGE('',*,*,#16264,.T.) ;
#22021=ORIENTED_EDGE('',*,*,#16281,.T.) ;
#22022=ORIENTED_EDGE('',*,*,#16274,.T.) ;
#22023=ORIENTED_EDGE('',*,*,#16282,.T.) ;
#22024=ORIENTED_EDGE('',*,*,#16275,.F.) ;
#22025=ORIENTED_EDGE('',*,*,#16281,.F.) ;
#22026=ORIENTED_EDGE('',*,*,#16263,.F.) ;
#22027=ORIENTED_EDGE('',*,*,#16262,.F.) ;
#22028=ORIENTED_EDGE('',*,*,#16283,.F.) ;
#22029=ORIENTED_EDGE('',*,*,#16276,.F.) ;
#22030=ORIENTED_EDGE('',*,*,#16282,.F.) ;
#22031=ORIENTED_EDGE('',*,*,#16261,.F.) ;
#22032=ORIENTED_EDGE('',*,*,#16284,.T.) ;
#22033=ORIENTED_EDGE('',*,*,#16277,.F.) ;
#22034=ORIENTED_EDGE('',*,*,#16283,.T.) ;
#22035=ORIENTED_EDGE('',*,*,#16260,.F.) ;
#22036=ORIENTED_EDGE('',*,*,#16269,.F.) ;
#22037=ORIENTED_EDGE('',*,*,#16278,.F.) ;
#22038=ORIENTED_EDGE('',*,*,#16284,.F.) ;
#22039=ORIENTED_EDGE('',*,*,#16285,.T.) ;
#22040=ORIENTED_EDGE('',*,*,#16286,.T.) ;
#22041=ORIENTED_EDGE('',*,*,#16287,.T.) ;
#22042=ORIENTED_EDGE('',*,*,#16288,.T.) ;
#22043=ORIENTED_EDGE('',*,*,#16287,.F.) ;
#22044=ORIENTED_EDGE('',*,*,#16289,.F.) ;
#22045=ORIENTED_EDGE('',*,*,#16285,.F.) ;
#22046=ORIENTED_EDGE('',*,*,#16290,.F.) ;
#22047=ORIENTED_EDGE('',*,*,#16288,.F.) ;
#22048=ORIENTED_EDGE('',*,*,#16290,.T.) ;
#22049=ORIENTED_EDGE('',*,*,#16286,.F.) ;
#22050=ORIENTED_EDGE('',*,*,#16289,.T.) ;
#22051=ORIENTED_EDGE('',*,*,#16291,.F.) ;
#22052=ORIENTED_EDGE('',*,*,#16292,.F.) ;
#22053=ORIENTED_EDGE('',*,*,#16293,.F.) ;
#22054=ORIENTED_EDGE('',*,*,#16294,.F.) ;
#22055=ORIENTED_EDGE('',*,*,#16295,.F.) ;
#22056=ORIENTED_EDGE('',*,*,#16292,.T.) ;
#22057=ORIENTED_EDGE('',*,*,#16293,.T.) ;
#22058=ORIENTED_EDGE('',*,*,#16291,.T.) ;
#22059=ORIENTED_EDGE('',*,*,#16295,.T.) ;
#22060=ORIENTED_EDGE('',*,*,#16296,.F.) ;
#22061=ORIENTED_EDGE('',*,*,#16297,.T.) ;
#22062=ORIENTED_EDGE('',*,*,#16298,.F.) ;
#22063=ORIENTED_EDGE('',*,*,#16299,.T.) ;
#22064=ORIENTED_EDGE('',*,*,#16300,.T.) ;
#22065=ORIENTED_EDGE('',*,*,#16301,.T.) ;
#22066=ORIENTED_EDGE('',*,*,#16302,.F.) ;
#22067=ORIENTED_EDGE('',*,*,#16303,.T.) ;
#22068=ORIENTED_EDGE('',*,*,#16304,.F.) ;
#22069=ORIENTED_EDGE('',*,*,#16300,.F.) ;
#22070=ORIENTED_EDGE('',*,*,#16305,.F.) ;
#22071=ORIENTED_EDGE('',*,*,#16299,.F.) ;
#22072=ORIENTED_EDGE('',*,*,#16306,.F.) ;
#22073=ORIENTED_EDGE('',*,*,#16301,.F.) ;
#22074=ORIENTED_EDGE('',*,*,#16305,.T.) ;
#22075=ORIENTED_EDGE('',*,*,#16306,.T.) ;
#22076=ORIENTED_EDGE('',*,*,#16298,.T.) ;
#22077=ORIENTED_EDGE('',*,*,#16307,.T.) ;
#22078=ORIENTED_EDGE('',*,*,#16302,.T.) ;
#22079=ORIENTED_EDGE('',*,*,#16294,.T.) ;
#22080=ORIENTED_EDGE('',*,*,#16304,.T.) ;
#22081=ORIENTED_EDGE('',*,*,#16308,.T.) ;
#22082=ORIENTED_EDGE('',*,*,#16296,.T.) ;
#22083=ORIENTED_EDGE('',*,*,#16297,.F.) ;
#22084=ORIENTED_EDGE('',*,*,#16308,.F.) ;
#22085=ORIENTED_EDGE('',*,*,#16303,.F.) ;
#22086=ORIENTED_EDGE('',*,*,#16307,.F.) ;
#26735=CYLINDRICAL_SURFACE('',#29922,0.65) ;
#26736=CYLINDRICAL_SURFACE('',#29925,0.65) ;
#26737=CYLINDRICAL_SURFACE('',#29928,0.65) ;
#26738=CYLINDRICAL_SURFACE('',#29931,0.65) ;
#26739=CYLINDRICAL_SURFACE('',#29934,0.65) ;
#26740=CYLINDRICAL_SURFACE('',#29937,0.65) ;
#26741=CYLINDRICAL_SURFACE('',#29940,3.) ;
#26742=CYLINDRICAL_SURFACE('',#29950,0.65) ;
#26743=CYLINDRICAL_SURFACE('',#29953,0.65) ;
#26744=CYLINDRICAL_SURFACE('',#29956,3.) ;
#26745=CYLINDRICAL_SURFACE('',#29966,1.28) ;
#26746=CYLINDRICAL_SURFACE('',#29969,1.28) ;
#26747=CYLINDRICAL_SURFACE('',#29972,1.2) ;
#26748=CYLINDRICAL_SURFACE('',#29975,1.5) ;
#26749=CYLINDRICAL_SURFACE('',#29981,1.2) ;
#26750=CYLINDRICAL_SURFACE('',#29984,1.5) ;
#26751=CYLINDRICAL_SURFACE('',#30048,3.) ;
#26752=CYLINDRICAL_SURFACE('',#30049,3.) ;
#26753=CYLINDRICAL_SURFACE('',#30050,2.6) ;
#26754=CYLINDRICAL_SURFACE('',#30051,2.6) ;
#26755=CYLINDRICAL_SURFACE('',#30074,1.5) ;
#26756=CYLINDRICAL_SURFACE('',#30076,1.2) ;
#26757=CYLINDRICAL_SURFACE('',#30082,1.5) ;
#26758=CYLINDRICAL_SURFACE('',#30083,1.2) ;
#26759=CYLINDRICAL_SURFACE('',#30084,3.) ;
#26760=CYLINDRICAL_SURFACE('',#30106,3.) ;
#26761=CYLINDRICAL_SURFACE('',#30121,3.) ;
#26762=CYLINDRICAL_SURFACE('',#30127,2.6) ;
#26763=CYLINDRICAL_SURFACE('',#30134,3.) ;
#26764=CYLINDRICAL_SURFACE('',#30140,3.) ;
#26765=CYLINDRICAL_SURFACE('',#30148,3.) ;
#26766=CYLINDRICAL_SURFACE('',#30153,3.) ;
#26767=CYLINDRICAL_SURFACE('',#30157,3.) ;
#26768=CYLINDRICAL_SURFACE('',#30167,3.) ;
#26769=CYLINDRICAL_SURFACE('',#30175,2.6) ;
#26770=CYLINDRICAL_SURFACE('',#30176,2.6) ;
#26771=CYLINDRICAL_SURFACE('',#30187,2.6) ;
#26772=CYLINDRICAL_SURFACE('',#30188,2.6) ;
#26773=CYLINDRICAL_SURFACE('',#30197,2.6) ;
#26774=CYLINDRICAL_SURFACE('',#30226,2.6) ;
#26775=CYLINDRICAL_SURFACE('',#30235,2.6) ;
#27510=ADVANCED_FACE('',(#2775),#26735,.F.) ;
#27511=ADVANCED_FACE('',(#2776),#26736,.F.) ;
#27512=ADVANCED_FACE('',(#2777),#26737,.F.) ;
#27513=ADVANCED_FACE('',(#2778),#26738,.F.) ;
#27514=ADVANCED_FACE('',(#2779),#26739,.F.) ;
#27515=ADVANCED_FACE('',(#2780),#26740,.F.) ;
#27516=ADVANCED_FACE('',(#2781),#26741,.T.) ;
#27517=ADVANCED_FACE('',(#2782),#1729,.T.) ;
#27518=ADVANCED_FACE('',(#2783),#1730,.T.) ;
#27519=ADVANCED_FACE('',(#2784),#1731,.T.) ;
#27520=ADVANCED_FACE('',(#2785,#1234,#1235),#1732,.T.) ;
#27521=ADVANCED_FACE('',(#2786,#1236,#1237),#1733,.F.) ;
#27522=ADVANCED_FACE('',(#2787),#1734,.T.) ;
#27523=ADVANCED_FACE('',(#2788),#1735,.T.) ;
#27524=ADVANCED_FACE('',(#2789),#26742,.F.) ;
#27525=ADVANCED_FACE('',(#2790),#26743,.F.) ;
#27526=ADVANCED_FACE('',(#2791),#26744,.T.) ;
#27527=ADVANCED_FACE('',(#2792),#1736,.T.) ;
#27528=ADVANCED_FACE('',(#2793),#1737,.T.) ;
#27529=ADVANCED_FACE('',(#2794),#1738,.T.) ;
#27530=ADVANCED_FACE('',(#2795,#1238,#1239),#1739,.T.) ;
#27531=ADVANCED_FACE('',(#2796,#1240,#1241),#1740,.F.) ;
#27532=ADVANCED_FACE('',(#2797),#1741,.T.) ;
#27533=ADVANCED_FACE('',(#2798),#1742,.T.) ;
#27534=ADVANCED_FACE('',(#2799),#26745,.F.) ;
#27535=ADVANCED_FACE('',(#2800),#26746,.F.) ;
#27536=ADVANCED_FACE('',(#2801),#26747,.F.) ;
#27537=ADVANCED_FACE('',(#2802),#26748,.T.) ;
#27538=ADVANCED_FACE('',(#2803,#1242),#1743,.T.) ;
#27539=ADVANCED_FACE('',(#2804,#1243,#1244,#1245,#1246),#1744,.T.) ;
#27540=ADVANCED_FACE('',(#2805),#26749,.F.) ;
#27541=ADVANCED_FACE('',(#2806),#26750,.T.) ;
#27542=ADVANCED_FACE('',(#2807,#1247),#1745,.T.) ;
#27543=ADVANCED_FACE('',(#2808),#1746,.T.) ;
#27544=ADVANCED_FACE('',(#2809),#1747,.T.) ;
#27545=ADVANCED_FACE('',(#2810),#1748,.T.) ;
#27546=ADVANCED_FACE('',(#2811),#1749,.T.) ;
#27547=ADVANCED_FACE('',(#2812),#1750,.T.) ;
#27548=ADVANCED_FACE('',(#2813,#1248),#1751,.F.) ;
#27549=ADVANCED_FACE('',(#2814),#1752,.F.) ;
#27550=ADVANCED_FACE('',(#2815),#1753,.F.) ;
#27551=ADVANCED_FACE('',(#2816,#1249,#1250),#1754,.F.) ;
#27552=ADVANCED_FACE('',(#2817),#1755,.F.) ;
#27553=ADVANCED_FACE('',(#2818),#1756,.F.) ;
#27554=ADVANCED_FACE('',(#2819),#1757,.T.) ;
#27555=ADVANCED_FACE('',(#2820),#1758,.F.) ;
#27556=ADVANCED_FACE('',(#2821),#1759,.F.) ;
#27557=ADVANCED_FACE('',(#2822),#1760,.F.) ;
#27558=ADVANCED_FACE('',(#2823),#1761,.F.) ;
#27559=ADVANCED_FACE('',(#2824),#1762,.F.) ;
#27560=ADVANCED_FACE('',(#2825),#1763,.F.) ;
#27561=ADVANCED_FACE('',(#2826),#1764,.T.) ;
#27562=ADVANCED_FACE('',(#2827),#1765,.F.) ;
#27563=ADVANCED_FACE('',(#2828),#1766,.F.) ;
#27564=ADVANCED_FACE('',(#2829),#1767,.F.) ;
#27565=ADVANCED_FACE('',(#2830),#1768,.T.) ;
#27566=ADVANCED_FACE('',(#2831),#1769,.F.) ;
#27567=ADVANCED_FACE('',(#2832),#1770,.F.) ;
#27568=ADVANCED_FACE('',(#2833,#1251),#1771,.F.) ;
#27569=ADVANCED_FACE('',(#2834),#1772,.F.) ;
#27570=ADVANCED_FACE('',(#2835),#1773,.F.) ;
#27571=ADVANCED_FACE('',(#2836),#1774,.F.) ;
#27572=ADVANCED_FACE('',(#2837),#1775,.T.) ;
#27573=ADVANCED_FACE('',(#2838),#1776,.T.) ;
#27574=ADVANCED_FACE('',(#2839),#1777,.T.) ;
#27575=ADVANCED_FACE('',(#2840),#1778,.T.) ;
#27576=ADVANCED_FACE('',(#2841,#1252),#1779,.F.) ;
#27577=ADVANCED_FACE('',(#2842),#1780,.T.) ;
#27578=ADVANCED_FACE('',(#2843),#1781,.F.) ;
#27579=ADVANCED_FACE('',(#2844),#1782,.F.) ;
#27580=ADVANCED_FACE('',(#2845,#1253),#1783,.F.) ;
#27581=ADVANCED_FACE('',(#2846),#1784,.F.) ;
#27582=ADVANCED_FACE('',(#2847),#1785,.F.) ;
#27583=ADVANCED_FACE('',(#2848),#1786,.F.) ;
#27584=ADVANCED_FACE('',(#2849),#1787,.T.) ;
#27585=ADVANCED_FACE('',(#2850),#1788,.T.) ;
#27586=ADVANCED_FACE('',(#2851),#1789,.T.) ;
#27587=ADVANCED_FACE('',(#2852),#1790,.T.) ;
#27588=ADVANCED_FACE('',(#2853,#1254),#1791,.T.) ;
#27589=ADVANCED_FACE('',(#2854,#1255),#1792,.T.) ;
#27590=ADVANCED_FACE('',(#2855),#26751,.T.) ;
#27591=ADVANCED_FACE('',(#2856),#26752,.T.) ;
#27592=ADVANCED_FACE('',(#2857),#26753,.F.) ;
#27593=ADVANCED_FACE('',(#2858),#26754,.F.) ;
#27594=ADVANCED_FACE('',(#2859),#1793,.T.) ;
#27595=ADVANCED_FACE('',(#2860),#1794,.F.) ;
#27596=ADVANCED_FACE('',(#2861),#1795,.F.) ;
#27597=ADVANCED_FACE('',(#2862),#1796,.T.) ;
#27598=ADVANCED_FACE('',(#2863),#1797,.F.) ;
#27599=ADVANCED_FACE('',(#2864),#1798,.F.) ;
#27600=ADVANCED_FACE('',(#2865,#1256),#1799,.F.) ;
#27601=ADVANCED_FACE('',(#2866,#1257),#1800,.F.) ;
#27602=ADVANCED_FACE('',(#2867),#1801,.F.) ;
#27603=ADVANCED_FACE('',(#2868,#1258,#1259),#1802,.F.) ;
#27604=ADVANCED_FACE('',(#2869),#1803,.F.) ;
#27605=ADVANCED_FACE('',(#2870),#1804,.F.) ;
#27606=ADVANCED_FACE('',(#2871,#1260),#1805,.F.) ;
#27607=ADVANCED_FACE('',(#2872),#1806,.T.) ;
#27608=ADVANCED_FACE('',(#2873),#1807,.T.) ;
#27609=ADVANCED_FACE('',(#2874),#1808,.T.) ;
#27610=ADVANCED_FACE('',(#2875),#1809,.T.) ;
#27611=ADVANCED_FACE('',(#2876),#1810,.T.) ;
#27612=ADVANCED_FACE('',(#2877,#1261),#1811,.T.) ;
#27613=ADVANCED_FACE('',(#2878),#26755,.T.) ;
#27614=ADVANCED_FACE('',(#2879),#26756,.F.) ;
#27615=ADVANCED_FACE('',(#2880,#1262,#1263,#1264,#1265),#1812,.T.) ;
#27616=ADVANCED_FACE('',(#2881,#1266),#1813,.T.) ;
#27617=ADVANCED_FACE('',(#2882),#26757,.T.) ;
#27618=ADVANCED_FACE('',(#2883),#26758,.F.) ;
#27619=ADVANCED_FACE('',(#2884),#26759,.T.) ;
#27620=ADVANCED_FACE('',(#2885),#1814,.F.) ;
#27621=ADVANCED_FACE('',(#2886),#1815,.F.) ;
#27622=ADVANCED_FACE('',(#2887),#1816,.F.) ;
#27623=ADVANCED_FACE('',(#2888),#1817,.F.) ;
#27624=ADVANCED_FACE('',(#2889),#1818,.F.) ;
#27625=ADVANCED_FACE('',(#2890),#1819,.T.) ;
#27626=ADVANCED_FACE('',(#2891),#1820,.F.) ;
#27627=ADVANCED_FACE('',(#2892),#1821,.F.) ;
#27628=ADVANCED_FACE('',(#2893),#1822,.F.) ;
#27629=ADVANCED_FACE('',(#2894),#1823,.T.) ;
#27630=ADVANCED_FACE('',(#2895,#1267),#1824,.F.) ;
#27631=ADVANCED_FACE('',(#2896),#1825,.F.) ;
#27632=ADVANCED_FACE('',(#2897),#1826,.F.) ;
#27633=ADVANCED_FACE('',(#2898,#1268),#1827,.F.) ;
#27634=ADVANCED_FACE('',(#2899),#1828,.F.) ;
#27635=ADVANCED_FACE('',(#2900),#1829,.T.) ;
#27636=ADVANCED_FACE('',(#2901,#1269),#1830,.F.) ;
#27637=ADVANCED_FACE('',(#2902),#1831,.F.) ;
#27638=ADVANCED_FACE('',(#2903),#26760,.T.) ;
#27639=ADVANCED_FACE('',(#2904),#1832,.T.) ;
#27640=ADVANCED_FACE('',(#2905),#1833,.T.) ;
#27641=ADVANCED_FACE('',(#2906),#1834,.T.) ;
#27642=ADVANCED_FACE('',(#2907),#1835,.T.) ;
#27643=ADVANCED_FACE('',(#2908),#1836,.F.) ;
#27644=ADVANCED_FACE('',(#2909),#1837,.F.) ;
#27645=ADVANCED_FACE('',(#2910),#1838,.T.) ;
#27646=ADVANCED_FACE('',(#2911),#1839,.T.) ;
#27647=ADVANCED_FACE('',(#2912),#1840,.T.) ;
#27648=ADVANCED_FACE('',(#2913),#1841,.T.) ;
#27649=ADVANCED_FACE('',(#2914),#26761,.T.) ;
#27650=ADVANCED_FACE('',(#2915),#1842,.T.) ;
#27651=ADVANCED_FACE('',(#2916),#1843,.T.) ;
#27652=ADVANCED_FACE('',(#2917),#1844,.T.) ;
#27653=ADVANCED_FACE('',(#2918),#26762,.F.) ;
#27654=ADVANCED_FACE('',(#2919),#1845,.T.) ;
#27655=ADVANCED_FACE('',(#2920),#1846,.T.) ;
#27656=ADVANCED_FACE('',(#2921),#1847,.F.) ;
#27657=ADVANCED_FACE('',(#2922),#1848,.F.) ;
#27658=ADVANCED_FACE('',(#2923),#26763,.T.) ;
#27659=ADVANCED_FACE('',(#2924),#1849,.T.) ;
#27660=ADVANCED_FACE('',(#2925),#1850,.T.) ;
#27661=ADVANCED_FACE('',(#2926),#1851,.T.) ;
#27662=ADVANCED_FACE('',(#2927),#26764,.T.) ;
#27663=ADVANCED_FACE('',(#2928),#1852,.T.) ;
#27664=ADVANCED_FACE('',(#2929),#1853,.T.) ;
#27665=ADVANCED_FACE('',(#2930),#1854,.T.) ;
#27666=ADVANCED_FACE('',(#2931),#1855,.F.) ;
#27667=ADVANCED_FACE('',(#2932),#1856,.F.) ;
#27668=ADVANCED_FACE('',(#2933),#26765,.T.) ;
#27669=ADVANCED_FACE('',(#2934),#1857,.T.) ;
#27670=ADVANCED_FACE('',(#2935),#1858,.T.) ;
#27671=ADVANCED_FACE('',(#2936),#26766,.T.) ;
#27672=ADVANCED_FACE('',(#2937),#1859,.T.) ;
#27673=ADVANCED_FACE('',(#2938),#1860,.T.) ;
#27674=ADVANCED_FACE('',(#2939),#1861,.T.) ;
#27675=ADVANCED_FACE('',(#2940),#26767,.T.) ;
#27676=ADVANCED_FACE('',(#2941),#1862,.T.) ;
#27677=ADVANCED_FACE('',(#2942),#1863,.T.) ;
#27678=ADVANCED_FACE('',(#2943),#1864,.T.) ;
#27679=ADVANCED_FACE('',(#2944),#1865,.T.) ;
#27680=ADVANCED_FACE('',(#2945),#1866,.T.) ;
#27681=ADVANCED_FACE('',(#2946),#26768,.T.) ;
#27682=ADVANCED_FACE('',(#2947),#1867,.T.) ;
#27683=ADVANCED_FACE('',(#2948),#1868,.T.) ;
#27684=ADVANCED_FACE('',(#2949),#1869,.F.) ;
#27685=ADVANCED_FACE('',(#2950),#1870,.T.) ;
#27686=ADVANCED_FACE('',(#2951),#1871,.T.) ;
#27687=ADVANCED_FACE('',(#2952),#26769,.F.) ;
#27688=ADVANCED_FACE('',(#2953),#26770,.F.) ;
#27689=ADVANCED_FACE('',(#2954),#1872,.T.) ;
#27690=ADVANCED_FACE('',(#2955),#1873,.T.) ;
#27691=ADVANCED_FACE('',(#2956),#1874,.F.) ;
#27692=ADVANCED_FACE('',(#2957),#1875,.T.) ;
#27693=ADVANCED_FACE('',(#2958),#1876,.T.) ;
#27694=ADVANCED_FACE('',(#2959),#1877,.T.) ;
#27695=ADVANCED_FACE('',(#2960),#26771,.F.) ;
#27696=ADVANCED_FACE('',(#2961),#26772,.F.) ;
#27697=ADVANCED_FACE('',(#2962),#1878,.F.) ;
#27698=ADVANCED_FACE('',(#2963),#1879,.F.) ;
#27699=ADVANCED_FACE('',(#2964),#1880,.F.) ;
#27700=ADVANCED_FACE('',(#2965),#1881,.T.) ;
#27701=ADVANCED_FACE('',(#2966),#1882,.T.) ;
#27702=ADVANCED_FACE('',(#2967),#26773,.F.) ;
#27703=ADVANCED_FACE('',(#2968),#1883,.T.) ;
#27704=ADVANCED_FACE('',(#2969),#1884,.T.) ;
#27705=ADVANCED_FACE('',(#2970),#1885,.T.) ;
#27706=ADVANCED_FACE('',(#2971),#1886,.T.) ;
#27707=ADVANCED_FACE('',(#2972),#1887,.T.) ;
#27708=ADVANCED_FACE('',(#2973),#1888,.T.) ;
#27709=ADVANCED_FACE('',(#2974),#1889,.F.) ;
#27710=ADVANCED_FACE('',(#2975),#1890,.F.) ;
#27711=ADVANCED_FACE('',(#2976),#1891,.T.) ;
#27712=ADVANCED_FACE('',(#2977),#1892,.T.) ;
#27713=ADVANCED_FACE('',(#2978),#1893,.T.) ;
#27714=ADVANCED_FACE('',(#2979),#1894,.T.) ;
#27715=ADVANCED_FACE('',(#2980),#1895,.T.) ;
#27716=ADVANCED_FACE('',(#2981),#1896,.F.) ;
#27717=ADVANCED_FACE('',(#2982),#1897,.F.) ;
#27718=ADVANCED_FACE('',(#2983),#1898,.F.) ;
#27719=ADVANCED_FACE('',(#2984),#1899,.T.) ;
#27720=ADVANCED_FACE('',(#2985),#1900,.F.) ;
#27721=ADVANCED_FACE('',(#2986),#1901,.F.) ;
#27722=ADVANCED_FACE('',(#2987),#1902,.T.) ;
#27723=ADVANCED_FACE('',(#2988),#1903,.T.) ;
#27724=ADVANCED_FACE('',(#2989),#1904,.F.) ;
#27725=ADVANCED_FACE('',(#2990),#1905,.F.) ;
#27726=ADVANCED_FACE('',(#2991),#1906,.F.) ;
#27727=ADVANCED_FACE('',(#2992),#1907,.F.) ;
#27728=ADVANCED_FACE('',(#2993),#1908,.F.) ;
#27729=ADVANCED_FACE('',(#2994),#1909,.F.) ;
#27730=ADVANCED_FACE('',(#2995),#26774,.F.) ;
#27731=ADVANCED_FACE('',(#2996),#1910,.T.) ;
#27732=ADVANCED_FACE('',(#2997),#1911,.T.) ;
#27733=ADVANCED_FACE('',(#2998),#1912,.T.) ;
#27734=ADVANCED_FACE('',(#2999),#1913,.F.) ;
#27735=ADVANCED_FACE('',(#3000),#1914,.F.) ;
#27736=ADVANCED_FACE('',(#3001),#26775,.F.) ;
#27737=ADVANCED_FACE('',(#3002),#1915,.F.) ;
#27738=ADVANCED_FACE('',(#3003),#1916,.F.) ;
#27739=ADVANCED_FACE('',(#3004),#1917,.F.) ;
#27740=ADVANCED_FACE('',(#3005),#1918,.F.) ;
#27741=ADVANCED_FACE('',(#3006),#1919,.T.) ;
#28634=CLOSED_SHELL('',(#27510,#27511,#27512,#27513,#27514,#27515,#27516,
#27517,#27518,#27519,#27520,#27521,#27522,#27523,#27524,#27525,#27526,#27527,
#27528,#27529,#27530,#27531,#27532,#27533,#27534,#27535,#27536,#27537,#27538,
#27539,#27540,#27541,#27542,#27543,#27544,#27545,#27546,#27547,#27548,#27549,
#27550,#27551,#27552,#27553,#27554,#27555,#27556,#27557,#27558,#27559,#27560,
#27561,#27562,#27563,#27564,#27565,#27566,#27567,#27568,#27569,#27570,#27571,
#27572,#27573,#27574,#27575,#27576,#27577,#27578,#27579,#27580,#27581,#27582,
#27583,#27584,#27585,#27586,#27587,#27588,#27589,#27590,#27591,#27592,#27593,
#27594,#27595,#27596,#27597,#27598,#27599,#27600,#27601,#27602,#27603,#27604,
#27605,#27606,#27607,#27608,#27609,#27610,#27611,#27612,#27613,#27614,#27615,
#27616,#27617,#27618,#27619,#27620,#27621,#27622,#27623,#27624,#27625,#27626,
#27627,#27628,#27629,#27630,#27631,#27632,#27633,#27634,#27635,#27636,#27637)) ;
#28635=CLOSED_SHELL('',(#27638,#27639,#27640,#27641,#27642,#27643)) ;
#28636=CLOSED_SHELL('',(#27644,#27645,#27646,#27647,#27648,#27649)) ;
#28637=CLOSED_SHELL('',(#27650,#27651,#27652,#27653)) ;
#28638=CLOSED_SHELL('',(#27654,#27655,#27656,#27657,#27658)) ;
#28639=CLOSED_SHELL('',(#27659,#27660,#27661,#27662,#27663)) ;
#28640=CLOSED_SHELL('',(#27664,#27665,#27666,#27667,#27668)) ;
#28641=CLOSED_SHELL('',(#27669,#27670,#27671,#27672,#27673)) ;
#28642=CLOSED_SHELL('',(#27674,#27675,#27676,#27677,#27678)) ;
#28643=CLOSED_SHELL('',(#27679,#27680,#27681,#27682,#27683)) ;
#28644=CLOSED_SHELL('',(#27684,#27685,#27686,#27687)) ;
#28645=CLOSED_SHELL('',(#27688,#27689,#27690,#27691)) ;
#28646=CLOSED_SHELL('',(#27692,#27693,#27694,#27695)) ;
#28647=CLOSED_SHELL('',(#27696,#27697,#27698,#27699)) ;
#28648=CLOSED_SHELL('',(#27700,#27701,#27702,#27703)) ;
#28649=CLOSED_SHELL('',(#27704,#27705,#27706,#27707,#27708,#27709)) ;
#28650=CLOSED_SHELL('',(#27710,#27711,#27712,#27713,#27714,#27715)) ;
#28651=CLOSED_SHELL('',(#27716,#27717,#27718,#27719,#27720,#27721,#27722,
#27723,#27724,#27725,#27726,#27727,#27728,#27729)) ;
#28652=CLOSED_SHELL('',(#27730,#27731,#27732,#27733)) ;
#28653=CLOSED_SHELL('',(#27734,#27735,#27736,#27737,#27738,#27739,#27740,
#27741)) ;
#29921=AXIS2_PLACEMENT_3D('',#43759,#34770,#34771) ;
#29922=AXIS2_PLACEMENT_3D('',#43760,#34772,#34773) ;
#29923=AXIS2_PLACEMENT_3D('',#43762,#34774,#34775) ;
#29924=AXIS2_PLACEMENT_3D('',#43765,#34777,#34778) ;
#29925=AXIS2_PLACEMENT_3D('',#43766,#34779,#34780) ;
#29926=AXIS2_PLACEMENT_3D('',#43768,#34781,#34782) ;
#29927=AXIS2_PLACEMENT_3D('',#43771,#34784,#34785) ;
#29928=AXIS2_PLACEMENT_3D('',#43772,#34786,#34787) ;
#29929=AXIS2_PLACEMENT_3D('',#43774,#34788,#34789) ;
#29930=AXIS2_PLACEMENT_3D('',#43777,#34791,#34792) ;
#29931=AXIS2_PLACEMENT_3D('',#43778,#34793,#34794) ;
#29932=AXIS2_PLACEMENT_3D('',#43780,#34795,#34796) ;
#29933=AXIS2_PLACEMENT_3D('',#43783,#34798,#34799) ;
#29934=AXIS2_PLACEMENT_3D('',#43784,#34800,#34801) ;
#29935=AXIS2_PLACEMENT_3D('',#43786,#34802,#34803) ;
#29936=AXIS2_PLACEMENT_3D('',#43789,#34805,#34806) ;
#29937=AXIS2_PLACEMENT_3D('',#43790,#34807,#34808) ;
#29938=AXIS2_PLACEMENT_3D('',#43792,#34809,#34810) ;
#29939=AXIS2_PLACEMENT_3D('',#43795,#34812,#34813) ;
#29940=AXIS2_PLACEMENT_3D('',#43796,#34814,#34815) ;
#29941=AXIS2_PLACEMENT_3D('',#43801,#34817,#34818) ;
#29942=AXIS2_PLACEMENT_3D('',#43804,#34820,#34821) ;
#29943=AXIS2_PLACEMENT_3D('',#43805,#34822,#34823) ;
#29944=AXIS2_PLACEMENT_3D('',#43814,#34828,#34829) ;
#29945=AXIS2_PLACEMENT_3D('',#43821,#34834,#34835) ;
#29946=AXIS2_PLACEMENT_3D('',#43827,#34839,#34840) ;
#29947=AXIS2_PLACEMENT_3D('',#43829,#34842,#34843) ;
#29948=AXIS2_PLACEMENT_3D('',#43831,#34845,#34846) ;
#29949=AXIS2_PLACEMENT_3D('',#43833,#34848,#34849) ;
#29950=AXIS2_PLACEMENT_3D('',#43834,#34850,#34851) ;
#29951=AXIS2_PLACEMENT_3D('',#43836,#34852,#34853) ;
#29952=AXIS2_PLACEMENT_3D('',#43839,#34855,#34856) ;
#29953=AXIS2_PLACEMENT_3D('',#43840,#34857,#34858) ;
#29954=AXIS2_PLACEMENT_3D('',#43842,#34859,#34860) ;
#29955=AXIS2_PLACEMENT_3D('',#43845,#34862,#34863) ;
#29956=AXIS2_PLACEMENT_3D('',#43846,#34864,#34865) ;
#29957=AXIS2_PLACEMENT_3D('',#43851,#34867,#34868) ;
#29958=AXIS2_PLACEMENT_3D('',#43854,#34870,#34871) ;
#29959=AXIS2_PLACEMENT_3D('',#43855,#34872,#34873) ;
#29960=AXIS2_PLACEMENT_3D('',#43864,#34878,#34879) ;
#29961=AXIS2_PLACEMENT_3D('',#43871,#34884,#34885) ;
#29962=AXIS2_PLACEMENT_3D('',#43877,#34889,#34890) ;
#29963=AXIS2_PLACEMENT_3D('',#43879,#34892,#34893) ;
#29964=AXIS2_PLACEMENT_3D('',#43881,#34895,#34896) ;
#29965=AXIS2_PLACEMENT_3D('',#43883,#34898,#34899) ;
#29966=AXIS2_PLACEMENT_3D('',#43884,#34900,#34901) ;
#29967=AXIS2_PLACEMENT_3D('',#43886,#34902,#34903) ;
#29968=AXIS2_PLACEMENT_3D('',#43889,#34905,#34906) ;
#29969=AXIS2_PLACEMENT_3D('',#43890,#34907,#34908) ;
#29970=AXIS2_PLACEMENT_3D('',#43892,#34909,#34910) ;
#29971=AXIS2_PLACEMENT_3D('',#43895,#34912,#34913) ;
#29972=AXIS2_PLACEMENT_3D('',#43896,#34914,#34915) ;
#29973=AXIS2_PLACEMENT_3D('',#43898,#34916,#34917) ;
#29974=AXIS2_PLACEMENT_3D('',#43901,#34919,#34920) ;
#29975=AXIS2_PLACEMENT_3D('',#43902,#34921,#34922) ;
#29976=AXIS2_PLACEMENT_3D('',#43904,#34923,#34924) ;
#29977=AXIS2_PLACEMENT_3D('',#43907,#34926,#34927) ;
#29978=AXIS2_PLACEMENT_3D('',#43908,#34928,#34929) ;
#29979=AXIS2_PLACEMENT_3D('',#43909,#34930,#34931) ;
#29980=AXIS2_PLACEMENT_3D('',#43921,#34937,#34938) ;
#29981=AXIS2_PLACEMENT_3D('',#43922,#34939,#34940) ;
#29982=AXIS2_PLACEMENT_3D('',#43924,#34941,#34942) ;
#29983=AXIS2_PLACEMENT_3D('',#43927,#34944,#34945) ;
#29984=AXIS2_PLACEMENT_3D('',#43928,#34946,#34947) ;
#29985=AXIS2_PLACEMENT_3D('',#43930,#34948,#34949) ;
#29986=AXIS2_PLACEMENT_3D('',#43932,#34951,#34952) ;
#29987=AXIS2_PLACEMENT_3D('',#43933,#34953,#34954) ;
#29988=AXIS2_PLACEMENT_3D('',#43934,#34955,#34956) ;
#29989=AXIS2_PLACEMENT_3D('',#43943,#34961,#34962) ;
#29990=AXIS2_PLACEMENT_3D('',#43949,#34966,#34967) ;
#29991=AXIS2_PLACEMENT_3D('',#43955,#34971,#34972) ;
#29992=AXIS2_PLACEMENT_3D('',#43958,#34975,#34976) ;
#29993=AXIS2_PLACEMENT_3D('',#43967,#34981,#34982) ;
#29994=AXIS2_PLACEMENT_3D('',#43973,#34986,#34987) ;
#29995=AXIS2_PLACEMENT_3D('',#43979,#34991,#34992) ;
#29996=AXIS2_PLACEMENT_3D('',#43987,#34997,#34998) ;
#29997=AXIS2_PLACEMENT_3D('',#43988,#34999,#35000) ;
#29998=AXIS2_PLACEMENT_3D('',#43997,#35005,#35006) ;
#29999=AXIS2_PLACEMENT_3D('',#43999,#35007,#35008) ;
#30000=AXIS2_PLACEMENT_3D('',#44000,#35009,#35010) ;
#30001=AXIS2_PLACEMENT_3D('',#44009,#35015,#35016) ;
#30002=AXIS2_PLACEMENT_3D('',#44011,#35017,#35018) ;
#30003=AXIS2_PLACEMENT_3D('',#44024,#35026,#35027) ;
#30004=AXIS2_PLACEMENT_3D('',#44038,#35035,#35036) ;
#30005=AXIS2_PLACEMENT_3D('',#44040,#35038,#35039) ;
#30006=AXIS2_PLACEMENT_3D('',#44044,#35041,#35042) ;
#30007=AXIS2_PLACEMENT_3D('',#44048,#35045,#35046) ;
#30008=AXIS2_PLACEMENT_3D('',#44053,#35049,#35050) ;
#30009=AXIS2_PLACEMENT_3D('',#44054,#35051,#35052) ;
#30010=AXIS2_PLACEMENT_3D('',#44060,#35056,#35057) ;
#30011=AXIS2_PLACEMENT_3D('',#44069,#35062,#35063) ;
#30012=AXIS2_PLACEMENT_3D('',#44078,#35068,#35069) ;
#30013=AXIS2_PLACEMENT_3D('',#44087,#35074,#35075) ;
#30014=AXIS2_PLACEMENT_3D('',#44093,#35079,#35080) ;
#30015=AXIS2_PLACEMENT_3D('',#44101,#35084,#35085) ;
#30016=AXIS2_PLACEMENT_3D('',#44102,#35086,#35087) ;
#30017=AXIS2_PLACEMENT_3D('',#44108,#35091,#35092) ;
#30018=AXIS2_PLACEMENT_3D('',#44109,#35093,#35094) ;
#30019=AXIS2_PLACEMENT_3D('',#44150,#35117,#35118) ;
#30020=AXIS2_PLACEMENT_3D('',#44152,#35119,#35120) ;
#30021=AXIS2_PLACEMENT_3D('',#44156,#35123,#35124) ;
#30022=AXIS2_PLACEMENT_3D('',#44160,#35127,#35128) ;
#30023=AXIS2_PLACEMENT_3D('',#44164,#35131,#35132) ;
#30024=AXIS2_PLACEMENT_3D('',#44170,#35136,#35137) ;
#30025=AXIS2_PLACEMENT_3D('',#44174,#35140,#35141) ;
#30026=AXIS2_PLACEMENT_3D('',#44180,#35145,#35146) ;
#30027=AXIS2_PLACEMENT_3D('',#44184,#35149,#35150) ;
#30028=AXIS2_PLACEMENT_3D('',#44189,#35154,#35155) ;
#30029=AXIS2_PLACEMENT_3D('',#44193,#35158,#35159) ;
#30030=AXIS2_PLACEMENT_3D('',#44195,#35160,#35161) ;
#30031=AXIS2_PLACEMENT_3D('',#44196,#35162,#35163) ;
#30032=AXIS2_PLACEMENT_3D('',#44198,#35164,#35165) ;
#30033=AXIS2_PLACEMENT_3D('',#44199,#35166,#35167) ;
#30034=AXIS2_PLACEMENT_3D('',#44206,#35172,#35173) ;
#30035=AXIS2_PLACEMENT_3D('',#44212,#35177,#35178) ;
#30036=AXIS2_PLACEMENT_3D('',#44215,#35181,#35182) ;
#30037=AXIS2_PLACEMENT_3D('',#44217,#35184,#35185) ;
#30038=AXIS2_PLACEMENT_3D('',#44218,#35186,#35187) ;
#30039=AXIS2_PLACEMENT_3D('',#44220,#35189,#35190) ;
#30040=AXIS2_PLACEMENT_3D('',#44221,#35191,#35192) ;
#30041=AXIS2_PLACEMENT_3D('',#44223,#35194,#35195) ;
#30042=AXIS2_PLACEMENT_3D('',#44224,#35196,#35197) ;
#30043=AXIS2_PLACEMENT_3D('',#44226,#35198,#35199) ;
#30044=AXIS2_PLACEMENT_3D('',#44228,#35200,#35201) ;
#30045=AXIS2_PLACEMENT_3D('',#44229,#35202,#35203) ;
#30046=AXIS2_PLACEMENT_3D('',#44231,#35204,#35205) ;
#30047=AXIS2_PLACEMENT_3D('',#44233,#35206,#35207) ;
#30048=AXIS2_PLACEMENT_3D('',#44234,#35208,#35209) ;
#30049=AXIS2_PLACEMENT_3D('',#44236,#35211,#35212) ;
#30050=AXIS2_PLACEMENT_3D('',#44238,#35214,#35215) ;
#30051=AXIS2_PLACEMENT_3D('',#44240,#35217,#35218) ;
#30052=AXIS2_PLACEMENT_3D('',#44242,#35220,#35221) ;
#30053=AXIS2_PLACEMENT_3D('',#44248,#35225,#35226) ;
#30054=AXIS2_PLACEMENT_3D('',#44257,#35231,#35232) ;
#30055=AXIS2_PLACEMENT_3D('',#44266,#35237,#35238) ;
#30056=AXIS2_PLACEMENT_3D('',#44269,#35241,#35242) ;
#30057=AXIS2_PLACEMENT_3D('',#44275,#35246,#35247) ;
#30058=AXIS2_PLACEMENT_3D('',#44278,#35250,#35251) ;
#30059=AXIS2_PLACEMENT_3D('',#44280,#35253,#35254) ;
#30060=AXIS2_PLACEMENT_3D('',#44282,#35256,#35257) ;
#30061=AXIS2_PLACEMENT_3D('',#44291,#35262,#35263) ;
#30062=AXIS2_PLACEMENT_3D('',#44294,#35266,#35267) ;
#30063=AXIS2_PLACEMENT_3D('',#44296,#35269,#35270) ;
#30064=AXIS2_PLACEMENT_3D('',#44298,#35272,#35273) ;
#30065=AXIS2_PLACEMENT_3D('',#44307,#35278,#35279) ;
#30066=AXIS2_PLACEMENT_3D('',#44310,#35282,#35283) ;
#30067=AXIS2_PLACEMENT_3D('',#44312,#35285,#35286) ;
#30068=AXIS2_PLACEMENT_3D('',#44314,#35288,#35289) ;
#30069=AXIS2_PLACEMENT_3D('',#44315,#35290,#35291) ;
#30070=AXIS2_PLACEMENT_3D('',#44317,#35292,#35293) ;
#30071=AXIS2_PLACEMENT_3D('',#44318,#35294,#35295) ;
#30072=AXIS2_PLACEMENT_3D('',#44320,#35296,#35297) ;
#30073=AXIS2_PLACEMENT_3D('',#44322,#35298,#35299) ;
#30074=AXIS2_PLACEMENT_3D('',#44323,#35300,#35301) ;
#30075=AXIS2_PLACEMENT_3D('',#44326,#35303,#35304) ;
#30076=AXIS2_PLACEMENT_3D('',#44327,#35305,#35306) ;
#30077=AXIS2_PLACEMENT_3D('',#44329,#35308,#35309) ;
#30078=AXIS2_PLACEMENT_3D('',#44331,#35310,#35311) ;
#30079=AXIS2_PLACEMENT_3D('',#44332,#35312,#35313) ;
#30080=AXIS2_PLACEMENT_3D('',#44334,#35314,#35315) ;
#30081=AXIS2_PLACEMENT_3D('',#44336,#35316,#35317) ;
#30082=AXIS2_PLACEMENT_3D('',#44337,#35318,#35319) ;
#30083=AXIS2_PLACEMENT_3D('',#44339,#35321,#35322) ;
#30084=AXIS2_PLACEMENT_3D('',#44341,#35324,#35325) ;
#30085=AXIS2_PLACEMENT_3D('',#44345,#35327,#35328) ;
#30086=AXIS2_PLACEMENT_3D('',#44346,#35329,#35330) ;
#30087=AXIS2_PLACEMENT_3D('',#44347,#35331,#35332) ;
#30088=AXIS2_PLACEMENT_3D('',#44348,#35333,#35334) ;
#30089=AXIS2_PLACEMENT_3D('',#44350,#35336,#35337) ;
#30090=AXIS2_PLACEMENT_3D('',#44352,#35339,#35340) ;
#30091=AXIS2_PLACEMENT_3D('',#44354,#35342,#35343) ;
#30092=AXIS2_PLACEMENT_3D('',#44360,#35347,#35348) ;
#30093=AXIS2_PLACEMENT_3D('',#44363,#35351,#35352) ;
#30094=AXIS2_PLACEMENT_3D('',#44364,#35353,#35354) ;
#30095=AXIS2_PLACEMENT_3D('',#44365,#35355,#35356) ;
#30096=AXIS2_PLACEMENT_3D('',#44367,#35358,#35359) ;
#30097=AXIS2_PLACEMENT_3D('',#44369,#35361,#35362) ;
#30098=AXIS2_PLACEMENT_3D('',#44373,#35365,#35366) ;
#30099=AXIS2_PLACEMENT_3D('',#44379,#35370,#35371) ;
#30100=AXIS2_PLACEMENT_3D('',#44388,#35376,#35377) ;
#30101=AXIS2_PLACEMENT_3D('',#44397,#35382,#35383) ;
#30102=AXIS2_PLACEMENT_3D('',#44401,#35387,#35388) ;
#30103=AXIS2_PLACEMENT_3D('',#44403,#35390,#35391) ;
#30104=AXIS2_PLACEMENT_3D('',#44405,#35393,#35394) ;
#30105=AXIS2_PLACEMENT_3D('',#44407,#35396,#35397) ;
#30106=AXIS2_PLACEMENT_3D('',#44408,#35398,#35399) ;
#30107=AXIS2_PLACEMENT_3D('',#44411,#35400,#35401) ;
#30108=AXIS2_PLACEMENT_3D('',#44415,#35403,#35404) ;
#30109=AXIS2_PLACEMENT_3D('',#44417,#35406,#35407) ;
#30110=AXIS2_PLACEMENT_3D('',#44423,#35411,#35412) ;
#30111=AXIS2_PLACEMENT_3D('',#44427,#35415,#35416) ;
#30112=AXIS2_PLACEMENT_3D('',#44431,#35419,#35420) ;
#30113=AXIS2_PLACEMENT_3D('',#44433,#35422,#35423) ;
#30114=AXIS2_PLACEMENT_3D('',#44434,#35424,#35425) ;
#30115=AXIS2_PLACEMENT_3D('',#44443,#35430,#35431) ;
#30116=AXIS2_PLACEMENT_3D('',#44446,#35432,#35433) ;
#30117=AXIS2_PLACEMENT_3D('',#44449,#35436,#35437) ;
#30118=AXIS2_PLACEMENT_3D('',#44453,#35440,#35441) ;
#30119=AXIS2_PLACEMENT_3D('',#44455,#35442,#35443) ;
#30120=AXIS2_PLACEMENT_3D('',#44457,#35445,#35446) ;
#30121=AXIS2_PLACEMENT_3D('',#44459,#35448,#35449) ;
#30122=AXIS2_PLACEMENT_3D('',#44460,#35450,#35451) ;
#30123=AXIS2_PLACEMENT_3D('',#44463,#35452,#35453) ;
#30124=AXIS2_PLACEMENT_3D('',#44465,#35455,#35456) ;
#30125=AXIS2_PLACEMENT_3D('',#44468,#35457,#35458) ;
#30126=AXIS2_PLACEMENT_3D('',#44470,#35460,#35461) ;
#30127=AXIS2_PLACEMENT_3D('',#44473,#35464,#35465) ;
#30128=AXIS2_PLACEMENT_3D('',#44474,#35466,#35467) ;
#30129=AXIS2_PLACEMENT_3D('',#44483,#35472,#35473) ;
#30130=AXIS2_PLACEMENT_3D('',#44489,#35477,#35478) ;
#30131=AXIS2_PLACEMENT_3D('',#44490,#35479,#35480) ;
#30132=AXIS2_PLACEMENT_3D('',#44491,#35481,#35482) ;
#30133=AXIS2_PLACEMENT_3D('',#44492,#35483,#35484) ;
#30134=AXIS2_PLACEMENT_3D('',#44493,#35485,#35486) ;
#30135=AXIS2_PLACEMENT_3D('',#44494,#35487,#35488) ;
#30136=AXIS2_PLACEMENT_3D('',#44499,#35490,#35491) ;
#30137=AXIS2_PLACEMENT_3D('',#44501,#35493,#35494) ;
#30138=AXIS2_PLACEMENT_3D('',#44507,#35498,#35499) ;
#30139=AXIS2_PLACEMENT_3D('',#44510,#35501,#35502) ;
#30140=AXIS2_PLACEMENT_3D('',#44511,#35503,#35504) ;
#30141=AXIS2_PLACEMENT_3D('',#44513,#35506,#35507) ;
#30142=AXIS2_PLACEMENT_3D('',#44514,#35508,#35509) ;
#30143=AXIS2_PLACEMENT_3D('',#44523,#35514,#35515) ;
#30144=AXIS2_PLACEMENT_3D('',#44529,#35519,#35520) ;
#30145=AXIS2_PLACEMENT_3D('',#44530,#35521,#35522) ;
#30146=AXIS2_PLACEMENT_3D('',#44531,#35523,#35524) ;
#30147=AXIS2_PLACEMENT_3D('',#44532,#35525,#35526) ;
#30148=AXIS2_PLACEMENT_3D('',#44533,#35527,#35528) ;
#30149=AXIS2_PLACEMENT_3D('',#44534,#35529,#35530) ;
#30150=AXIS2_PLACEMENT_3D('',#44540,#35533,#35534) ;
#30151=AXIS2_PLACEMENT_3D('',#44541,#35535,#35536) ;
#30152=AXIS2_PLACEMENT_3D('',#44546,#35538,#35539) ;
#30153=AXIS2_PLACEMENT_3D('',#44548,#35541,#35542) ;
#30154=AXIS2_PLACEMENT_3D('',#44551,#35545,#35546) ;
#30155=AXIS2_PLACEMENT_3D('',#44553,#35548,#35549) ;
#30156=AXIS2_PLACEMENT_3D('',#44554,#35550,#35551) ;
#30157=AXIS2_PLACEMENT_3D('',#44563,#35556,#35557) ;
#30158=AXIS2_PLACEMENT_3D('',#44565,#35558,#35559) ;
#30159=AXIS2_PLACEMENT_3D('',#44568,#35561,#35562) ;
#30160=AXIS2_PLACEMENT_3D('',#44569,#35563,#35564) ;
#30161=AXIS2_PLACEMENT_3D('',#44571,#35566,#35567) ;
#30162=AXIS2_PLACEMENT_3D('',#44573,#35569,#35570) ;
#30163=AXIS2_PLACEMENT_3D('',#44574,#35571,#35572) ;
#30164=AXIS2_PLACEMENT_3D('',#44580,#35575,#35576) ;
#30165=AXIS2_PLACEMENT_3D('',#44581,#35577,#35578) ;
#30166=AXIS2_PLACEMENT_3D('',#44586,#35580,#35581) ;
#30167=AXIS2_PLACEMENT_3D('',#44588,#35583,#35584) ;
#30168=AXIS2_PLACEMENT_3D('',#44591,#35587,#35588) ;
#30169=AXIS2_PLACEMENT_3D('',#44593,#35590,#35591) ;
#30170=AXIS2_PLACEMENT_3D('',#44594,#35592,#35593) ;
#30171=AXIS2_PLACEMENT_3D('',#44603,#35598,#35599) ;
#30172=AXIS2_PLACEMENT_3D('',#44604,#35600,#35601) ;
#30173=AXIS2_PLACEMENT_3D('',#44605,#35602,#35603) ;
#30174=AXIS2_PLACEMENT_3D('',#44606,#35604,#35605) ;
#30175=AXIS2_PLACEMENT_3D('',#44607,#35606,#35607) ;
#30176=AXIS2_PLACEMENT_3D('',#44608,#35608,#35609) ;
#30177=AXIS2_PLACEMENT_3D('',#44613,#35611,#35612) ;
#30178=AXIS2_PLACEMENT_3D('',#44616,#35614,#35615) ;
#30179=AXIS2_PLACEMENT_3D('',#44617,#35616,#35617) ;
#30180=AXIS2_PLACEMENT_3D('',#44619,#35619,#35620) ;
#30181=AXIS2_PLACEMENT_3D('',#44621,#35622,#35623) ;
#30182=AXIS2_PLACEMENT_3D('',#44622,#35624,#35625) ;
#30183=AXIS2_PLACEMENT_3D('',#44631,#35630,#35631) ;
#30184=AXIS2_PLACEMENT_3D('',#44632,#35632,#35633) ;
#30185=AXIS2_PLACEMENT_3D('',#44633,#35634,#35635) ;
#30186=AXIS2_PLACEMENT_3D('',#44634,#35636,#35637) ;
#30187=AXIS2_PLACEMENT_3D('',#44635,#35638,#35639) ;
#30188=AXIS2_PLACEMENT_3D('',#44636,#35640,#35641) ;
#30189=AXIS2_PLACEMENT_3D('',#44641,#35643,#35644) ;
#30190=AXIS2_PLACEMENT_3D('',#44644,#35646,#35647) ;
#30191=AXIS2_PLACEMENT_3D('',#44645,#35648,#35649) ;
#30192=AXIS2_PLACEMENT_3D('',#44647,#35651,#35652) ;
#30193=AXIS2_PLACEMENT_3D('',#44649,#35654,#35655) ;
#30194=AXIS2_PLACEMENT_3D('',#44650,#35656,#35657) ;
#30195=AXIS2_PLACEMENT_3D('',#44659,#35662,#35663) ;
#30196=AXIS2_PLACEMENT_3D('',#44660,#35664,#35665) ;
#30197=AXIS2_PLACEMENT_3D('',#44661,#35666,#35667) ;
#30198=AXIS2_PLACEMENT_3D('',#44662,#35668,#35669) ;
#30199=AXIS2_PLACEMENT_3D('',#44663,#35670,#35671) ;
#30200=AXIS2_PLACEMENT_3D('',#44664,#35672,#35673) ;
#30201=AXIS2_PLACEMENT_3D('',#44673,#35678,#35679) ;
#30202=AXIS2_PLACEMENT_3D('',#44679,#35683,#35684) ;
#30203=AXIS2_PLACEMENT_3D('',#44685,#35688,#35689) ;
#30204=AXIS2_PLACEMENT_3D('',#44688,#35692,#35693) ;
#30205=AXIS2_PLACEMENT_3D('',#44689,#35694,#35695) ;
#30206=AXIS2_PLACEMENT_3D('',#44690,#35696,#35697) ;
#30207=AXIS2_PLACEMENT_3D('',#44699,#35702,#35703) ;
#30208=AXIS2_PLACEMENT_3D('',#44708,#35708,#35709) ;
#30209=AXIS2_PLACEMENT_3D('',#44711,#35712,#35713) ;
#30210=AXIS2_PLACEMENT_3D('',#44713,#35715,#35716) ;
#30211=AXIS2_PLACEMENT_3D('',#44715,#35718,#35719) ;
#30212=AXIS2_PLACEMENT_3D('',#44716,#35720,#35721) ;
#30213=AXIS2_PLACEMENT_3D('',#44725,#35726,#35727) ;
#30214=AXIS2_PLACEMENT_3D('',#44731,#35731,#35732) ;
#30215=AXIS2_PLACEMENT_3D('',#44737,#35736,#35737) ;
#30216=AXIS2_PLACEMENT_3D('',#44755,#35747,#35748) ;
#30217=AXIS2_PLACEMENT_3D('',#44759,#35751,#35752) ;
#30218=AXIS2_PLACEMENT_3D('',#44763,#35755,#35756) ;
#30219=AXIS2_PLACEMENT_3D('',#44777,#35764,#35765) ;
#30220=AXIS2_PLACEMENT_3D('',#44780,#35768,#35769) ;
#30221=AXIS2_PLACEMENT_3D('',#44781,#35770,#35771) ;
#30222=AXIS2_PLACEMENT_3D('',#44783,#35773,#35774) ;
#30223=AXIS2_PLACEMENT_3D('',#44785,#35776,#35777) ;
#30224=AXIS2_PLACEMENT_3D('',#44787,#35779,#35780) ;
#30225=AXIS2_PLACEMENT_3D('',#44789,#35782,#35783) ;
#30226=AXIS2_PLACEMENT_3D('',#44790,#35784,#35785) ;
#30227=AXIS2_PLACEMENT_3D('',#44795,#35787,#35788) ;
#30228=AXIS2_PLACEMENT_3D('',#44798,#35790,#35791) ;
#30229=AXIS2_PLACEMENT_3D('',#44799,#35792,#35793) ;
#30230=AXIS2_PLACEMENT_3D('',#44802,#35796,#35797) ;
#30231=AXIS2_PLACEMENT_3D('',#44803,#35798,#35799) ;
#30232=AXIS2_PLACEMENT_3D('',#44804,#35800,#35801) ;
#30233=AXIS2_PLACEMENT_3D('',#44807,#35802,#35803) ;
#30234=AXIS2_PLACEMENT_3D('',#44809,#35805,#35806) ;
#30235=AXIS2_PLACEMENT_3D('',#44815,#35810,#35811) ;
#30236=AXIS2_PLACEMENT_3D('',#44817,#35812,#35813) ;
#30237=AXIS2_PLACEMENT_3D('',#44821,#35815,#35816) ;
#30238=AXIS2_PLACEMENT_3D('',#44825,#35818,#35819) ;
#30239=AXIS2_PLACEMENT_3D('',#44829,#35821,#35822) ;
#30240=AXIS2_PLACEMENT_3D('',#44832,#35824,#35825) ;
#30241=AXIS2_PLACEMENT_3D('',#44833,#35826,#35827) ;
#30242=AXIS2_PLACEMENT_3D('',#44835,#35829,#35830) ;
#30243=AXIS2_PLACEMENT_3D('',#44837,#35832,#35833) ;
#30244=AXIS2_PLACEMENT_3D('',#44839,#35835,#35836) ;
#30245=AXIS2_PLACEMENT_3D('',#44841,#35838,#35839) ;
#34770=DIRECTION('axis',(0.,0.,1.)) ;
#34771=DIRECTION('refdir',(1.,0.,0.)) ;
#34772=DIRECTION('center_axis',(0.,0.,1.)) ;
#34773=DIRECTION('ref_axis',(1.,0.,0.)) ;
#34774=DIRECTION('center_axis',(0.,0.,1.)) ;
#34775=DIRECTION('ref_axis',(1.,0.,0.)) ;
#34776=DIRECTION('',(0.,0.,1.)) ;
#34777=DIRECTION('center_axis',(0.,0.,-1.)) ;
#34778=DIRECTION('ref_axis',(1.,0.,0.)) ;
#34779=DIRECTION('center_axis',(0.,0.,1.)) ;
#34780=DIRECTION('ref_axis',(1.,0.,0.)) ;
#34781=DIRECTION('center_axis',(0.,0.,1.)) ;
#34782=DIRECTION('ref_axis',(1.,0.,0.)) ;
#34783=DIRECTION('',(0.,0.,1.)) ;
#34784=DIRECTION('center_axis',(0.,0.,-1.)) ;
#34785=DIRECTION('ref_axis',(1.,0.,0.)) ;
#34786=DIRECTION('center_axis',(0.,0.,1.)) ;
#34787=DIRECTION('ref_axis',(1.,0.,0.)) ;
#34788=DIRECTION('center_axis',(0.,0.,1.)) ;
#34789=DIRECTION('ref_axis',(1.,0.,0.)) ;
#34790=DIRECTION('',(0.,0.,1.)) ;
#34791=DIRECTION('center_axis',(0.,0.,-1.)) ;
#34792=DIRECTION('ref_axis',(1.,0.,0.)) ;
#34793=DIRECTION('center_axis',(0.,0.,1.)) ;
#34794=DIRECTION('ref_axis',(1.,0.,0.)) ;
#34795=DIRECTION('center_axis',(0.,0.,1.)) ;
#34796=DIRECTION('ref_axis',(1.,0.,0.)) ;
#34797=DIRECTION('',(0.,0.,1.)) ;
#34798=DIRECTION('center_axis',(0.,0.,-1.)) ;
#34799=DIRECTION('ref_axis',(1.,0.,0.)) ;
#34800=DIRECTION('center_axis',(0.,0.,1.)) ;
#34801=DIRECTION('ref_axis',(1.,0.,0.)) ;
#34802=DIRECTION('center_axis',(0.,0.,1.)) ;
#34803=DIRECTION('ref_axis',(1.,0.,0.)) ;
#34804=DIRECTION('',(0.,0.,1.)) ;
#34805=DIRECTION('center_axis',(0.,0.,-1.)) ;
#34806=DIRECTION('ref_axis',(1.,0.,0.)) ;
#34807=DIRECTION('center_axis',(0.,0.,1.)) ;
#34808=DIRECTION('ref_axis',(1.,0.,0.)) ;
#34809=DIRECTION('center_axis',(0.,0.,1.)) ;
#34810=DIRECTION('ref_axis',(1.,0.,0.)) ;
#34811=DIRECTION('',(0.,0.,1.)) ;
#34812=DIRECTION('center_axis',(0.,0.,-1.)) ;
#34813=DIRECTION('ref_axis',(1.,0.,0.)) ;
#34814=DIRECTION('center_axis',(0.,1.,0.)) ;
#34815=DIRECTION('ref_axis',(1.,0.,0.)) ;
#34816=DIRECTION('',(0.,-1.,0.)) ;
#34817=DIRECTION('center_axis',(0.,1.,0.)) ;
#34818=DIRECTION('ref_axis',(1.,0.,0.)) ;
#34819=DIRECTION('',(0.,1.,0.)) ;
#34820=DIRECTION('center_axis',(0.,-1.,0.)) ;
#34821=DIRECTION('ref_axis',(1.,0.,0.)) ;
#34822=DIRECTION('center_axis',(-1.,0.,0.)) ;
#34823=DIRECTION('ref_axis',(0.,0.,1.)) ;
#34824=DIRECTION('',(0.,0.,-1.)) ;
#34825=DIRECTION('',(0.,1.,0.)) ;
#34826=DIRECTION('',(0.,0.,-1.)) ;
#34827=DIRECTION('',(0.,-1.,0.)) ;
#34828=DIRECTION('center_axis',(0.,-1.,0.)) ;
#34829=DIRECTION('ref_axis',(0.,0.,-1.)) ;
#34830=DIRECTION('',(1.,0.,0.)) ;
#34831=DIRECTION('',(-1.,0.,0.)) ;
#34832=DIRECTION('',(0.,0.,-1.)) ;
#34833=DIRECTION('',(1.,0.,0.)) ;
#34834=DIRECTION('center_axis',(1.,0.,0.)) ;
#34835=DIRECTION('ref_axis',(0.,0.,-1.)) ;
#34836=DIRECTION('',(0.,-1.,0.)) ;
#34837=DIRECTION('',(0.,0.,-1.)) ;
#34838=DIRECTION('',(0.,1.,0.)) ;
#34839=DIRECTION('center_axis',(0.,0.,1.)) ;
#34840=DIRECTION('ref_axis',(1.,0.,0.)) ;
#34841=DIRECTION('',(-1.,0.,0.)) ;
#34842=DIRECTION('center_axis',(0.,0.,1.)) ;
#34843=DIRECTION('ref_axis',(1.,0.,0.)) ;
#34844=DIRECTION('',(1.,0.,0.)) ;
#34845=DIRECTION('center_axis',(0.,0.,1.)) ;
#34846=DIRECTION('ref_axis',(1.,0.,0.)) ;
#34847=DIRECTION('',(-1.,0.,0.)) ;
#34848=DIRECTION('center_axis',(0.,1.,0.)) ;
#34849=DIRECTION('ref_axis',(0.,0.,1.)) ;
#34850=DIRECTION('center_axis',(0.,0.,1.)) ;
#34851=DIRECTION('ref_axis',(1.,0.,0.)) ;
#34852=DIRECTION('center_axis',(0.,0.,1.)) ;
#34853=DIRECTION('ref_axis',(1.,0.,0.)) ;
#34854=DIRECTION('',(0.,0.,1.)) ;
#34855=DIRECTION('center_axis',(0.,0.,-1.)) ;
#34856=DIRECTION('ref_axis',(1.,0.,0.)) ;
#34857=DIRECTION('center_axis',(0.,0.,1.)) ;
#34858=DIRECTION('ref_axis',(1.,0.,0.)) ;
#34859=DIRECTION('center_axis',(0.,0.,1.)) ;
#34860=DIRECTION('ref_axis',(1.,0.,0.)) ;
#34861=DIRECTION('',(0.,0.,1.)) ;
#34862=DIRECTION('center_axis',(0.,0.,-1.)) ;
#34863=DIRECTION('ref_axis',(1.,0.,0.)) ;
#34864=DIRECTION('center_axis',(0.,1.,0.)) ;
#34865=DIRECTION('ref_axis',(1.,0.,0.)) ;
#34866=DIRECTION('',(0.,-1.,0.)) ;
#34867=DIRECTION('center_axis',(0.,1.,0.)) ;
#34868=DIRECTION('ref_axis',(1.,0.,0.)) ;
#34869=DIRECTION('',(0.,1.,0.)) ;
#34870=DIRECTION('center_axis',(0.,-1.,0.)) ;
#34871=DIRECTION('ref_axis',(1.,0.,0.)) ;
#34872=DIRECTION('center_axis',(-1.,0.,0.)) ;
#34873=DIRECTION('ref_axis',(0.,0.,1.)) ;
#34874=DIRECTION('',(0.,0.,-1.)) ;
#34875=DIRECTION('',(0.,1.,0.)) ;
#34876=DIRECTION('',(0.,0.,-1.)) ;
#34877=DIRECTION('',(0.,-1.,0.)) ;
#34878=DIRECTION('center_axis',(0.,-1.,0.)) ;
#34879=DIRECTION('ref_axis',(0.,0.,-1.)) ;
#34880=DIRECTION('',(1.,0.,0.)) ;
#34881=DIRECTION('',(-1.,0.,0.)) ;
#34882=DIRECTION('',(0.,0.,-1.)) ;
#34883=DIRECTION('',(1.,0.,0.)) ;
#34884=DIRECTION('center_axis',(1.,0.,0.)) ;
#34885=DIRECTION('ref_axis',(0.,0.,-1.)) ;
#34886=DIRECTION('',(0.,-1.,0.)) ;
#34887=DIRECTION('',(0.,0.,-1.)) ;
#34888=DIRECTION('',(0.,1.,0.)) ;
#34889=DIRECTION('center_axis',(0.,0.,1.)) ;
#34890=DIRECTION('ref_axis',(1.,0.,0.)) ;
#34891=DIRECTION('',(-1.,0.,0.)) ;
#34892=DIRECTION('center_axis',(0.,0.,1.)) ;
#34893=DIRECTION('ref_axis',(1.,0.,0.)) ;
#34894=DIRECTION('',(1.,0.,0.)) ;
#34895=DIRECTION('center_axis',(0.,0.,1.)) ;
#34896=DIRECTION('ref_axis',(1.,0.,0.)) ;
#34897=DIRECTION('',(-1.,0.,0.)) ;
#34898=DIRECTION('center_axis',(0.,1.,0.)) ;
#34899=DIRECTION('ref_axis',(0.,0.,1.)) ;
#34900=DIRECTION('center_axis',(0.,1.,0.)) ;
#34901=DIRECTION('ref_axis',(1.,0.,0.)) ;
#34902=DIRECTION('center_axis',(0.,1.,0.)) ;
#34903=DIRECTION('ref_axis',(1.,0.,0.)) ;
#34904=DIRECTION('',(0.,1.,0.)) ;
#34905=DIRECTION('center_axis',(0.,-1.,0.)) ;
#34906=DIRECTION('ref_axis',(1.,0.,0.)) ;
#34907=DIRECTION('center_axis',(0.,1.,0.)) ;
#34908=DIRECTION('ref_axis',(1.,0.,0.)) ;
#34909=DIRECTION('center_axis',(0.,1.,0.)) ;
#34910=DIRECTION('ref_axis',(1.,0.,0.)) ;
#34911=DIRECTION('',(0.,1.,0.)) ;
#34912=DIRECTION('center_axis',(0.,-1.,0.)) ;
#34913=DIRECTION('ref_axis',(1.,0.,0.)) ;
#34914=DIRECTION('center_axis',(0.,0.,1.)) ;
#34915=DIRECTION('ref_axis',(1.,0.,0.)) ;
#34916=DIRECTION('center_axis',(0.,0.,1.)) ;
#34917=DIRECTION('ref_axis',(1.,0.,0.)) ;
#34918=DIRECTION('',(0.,0.,1.)) ;
#34919=DIRECTION('center_axis',(0.,0.,-1.)) ;
#34920=DIRECTION('ref_axis',(1.,0.,0.)) ;
#34921=DIRECTION('center_axis',(0.,0.,1.)) ;
#34922=DIRECTION('ref_axis',(1.,0.,0.)) ;
#34923=DIRECTION('center_axis',(0.,0.,1.)) ;
#34924=DIRECTION('ref_axis',(1.,0.,0.)) ;
#34925=DIRECTION('',(0.,0.,-1.)) ;
#34926=DIRECTION('center_axis',(0.,0.,-1.)) ;
#34927=DIRECTION('ref_axis',(1.,0.,0.)) ;
#34928=DIRECTION('center_axis',(0.,0.,1.)) ;
#34929=DIRECTION('ref_axis',(1.,0.,0.)) ;
#34930=DIRECTION('center_axis',(0.,0.,1.)) ;
#34931=DIRECTION('ref_axis',(1.,0.,0.)) ;
#34932=DIRECTION('',(0.,1.,0.)) ;
#34933=DIRECTION('',(-1.,0.,0.)) ;
#34934=DIRECTION('',(0.,-1.,0.)) ;
#34935=DIRECTION('',(-1.,0.,0.)) ;
#34936=DIRECTION('',(1.,0.,0.)) ;
#34937=DIRECTION('center_axis',(0.,0.,-1.)) ;
#34938=DIRECTION('ref_axis',(1.,0.,0.)) ;
#34939=DIRECTION('center_axis',(0.,0.,1.)) ;
#34940=DIRECTION('ref_axis',(1.,0.,0.)) ;
#34941=DIRECTION('center_axis',(0.,0.,1.)) ;
#34942=DIRECTION('ref_axis',(1.,0.,0.)) ;
#34943=DIRECTION('',(0.,0.,1.)) ;
#34944=DIRECTION('center_axis',(0.,0.,-1.)) ;
#34945=DIRECTION('ref_axis',(1.,0.,0.)) ;
#34946=DIRECTION('center_axis',(0.,0.,1.)) ;
#34947=DIRECTION('ref_axis',(1.,0.,0.)) ;
#34948=DIRECTION('center_axis',(0.,0.,1.)) ;
#34949=DIRECTION('ref_axis',(1.,0.,0.)) ;
#34950=DIRECTION('',(0.,0.,-1.)) ;
#34951=DIRECTION('center_axis',(0.,0.,1.)) ;
#34952=DIRECTION('ref_axis',(1.,0.,0.)) ;
#34953=DIRECTION('center_axis',(0.,0.,1.)) ;
#34954=DIRECTION('ref_axis',(1.,0.,0.)) ;
#34955=DIRECTION('center_axis',(0.,-1.,0.)) ;
#34956=DIRECTION('ref_axis',(0.,0.,-1.)) ;
#34957=DIRECTION('',(1.,0.,0.)) ;
#34958=DIRECTION('',(0.,0.,-1.)) ;
#34959=DIRECTION('',(-1.,0.,0.)) ;
#34960=DIRECTION('',(0.,0.,-1.)) ;
#34961=DIRECTION('center_axis',(-1.,0.,0.)) ;
#34962=DIRECTION('ref_axis',(0.,0.,1.)) ;
#34963=DIRECTION('',(0.,-1.,0.)) ;
#34964=DIRECTION('',(0.,1.,0.)) ;
#34965=DIRECTION('',(0.,0.,-1.)) ;
#34966=DIRECTION('center_axis',(0.,1.,0.)) ;
#34967=DIRECTION('ref_axis',(0.,0.,1.)) ;
#34968=DIRECTION('',(-1.,0.,0.)) ;
#34969=DIRECTION('',(1.,0.,0.)) ;
#34970=DIRECTION('',(0.,0.,-1.)) ;
#34971=DIRECTION('center_axis',(1.,0.,0.)) ;
#34972=DIRECTION('ref_axis',(0.,0.,-1.)) ;
#34973=DIRECTION('',(0.,1.,0.)) ;
#34974=DIRECTION('',(0.,-1.,0.)) ;
#34975=DIRECTION('center_axis',(0.,0.,1.)) ;
#34976=DIRECTION('ref_axis',(1.,0.,0.)) ;
#34977=DIRECTION('',(0.,-1.,0.)) ;
#34978=DIRECTION('',(-1.,0.,0.)) ;
#34979=DIRECTION('',(0.,1.,0.)) ;
#34980=DIRECTION('',(1.,0.,0.)) ;
#34981=DIRECTION('center_axis',(1.,0.,0.)) ;
#34982=DIRECTION('ref_axis',(0.,0.,-1.)) ;
#34983=DIRECTION('',(0.,0.,-1.)) ;
#34984=DIRECTION('',(0.,0.,-1.)) ;
#34985=DIRECTION('',(0.,-1.,0.)) ;
#34986=DIRECTION('center_axis',(-1.,0.,0.)) ;
#34987=DIRECTION('ref_axis',(0.,0.,1.)) ;
#34988=DIRECTION('',(0.,0.,-1.)) ;
#34989=DIRECTION('',(0.,0.,-1.)) ;
#34990=DIRECTION('',(0.,1.,0.)) ;
#34991=DIRECTION('center_axis',(0.,0.,1.)) ;
#34992=DIRECTION('ref_axis',(1.,0.,0.)) ;
#34993=DIRECTION('',(-1.,0.,0.)) ;
#34994=DIRECTION('',(1.,0.,0.)) ;
#34995=DIRECTION('',(0.,-1.,0.)) ;
#34996=DIRECTION('',(1.,0.,0.)) ;
#34997=DIRECTION('center_axis',(0.,0.,1.)) ;
#34998=DIRECTION('ref_axis',(1.,0.,0.)) ;
#34999=DIRECTION('center_axis',(0.,0.,1.)) ;
#35000=DIRECTION('ref_axis',(1.,0.,0.)) ;
#35001=DIRECTION('',(0.,1.,0.)) ;
#35002=DIRECTION('',(-1.,0.,0.)) ;
#35003=DIRECTION('',(0.,1.,0.)) ;
#35004=DIRECTION('',(-1.,0.,0.)) ;
#35005=DIRECTION('center_axis',(0.,0.,1.)) ;
#35006=DIRECTION('ref_axis',(1.,0.,0.)) ;
#35007=DIRECTION('center_axis',(0.,0.,1.)) ;
#35008=DIRECTION('ref_axis',(1.,0.,0.)) ;
#35009=DIRECTION('center_axis',(0.,0.,1.)) ;
#35010=DIRECTION('ref_axis',(1.,0.,0.)) ;
#35011=DIRECTION('',(0.,1.,0.)) ;
#35012=DIRECTION('',(1.,0.,0.)) ;
#35013=DIRECTION('',(0.,-1.,0.)) ;
#35014=DIRECTION('',(-1.,0.,0.)) ;
#35015=DIRECTION('center_axis',(0.,1.,0.)) ;
#35016=DIRECTION('ref_axis',(0.,0.,1.)) ;
#35017=DIRECTION('center_axis',(0.,-1.,0.)) ;
#35018=DIRECTION('ref_axis',(1.,0.,0.)) ;
#35019=DIRECTION('',(-1.,0.,0.)) ;
#35020=DIRECTION('',(0.,0.,-1.)) ;
#35021=DIRECTION('',(-1.,0.,0.)) ;
#35022=DIRECTION('',(0.,0.,-1.)) ;
#35023=DIRECTION('',(0.,0.,-1.)) ;
#35024=DIRECTION('',(1.,0.,0.)) ;
#35025=DIRECTION('',(0.,0.,-1.)) ;
#35026=DIRECTION('center_axis',(0.,-1.,0.)) ;
#35027=DIRECTION('ref_axis',(0.,0.,-1.)) ;
#35028=DIRECTION('',(0.,0.,-1.)) ;
#35029=DIRECTION('',(-1.,0.,0.)) ;
#35030=DIRECTION('',(0.,0.,-1.)) ;
#35031=DIRECTION('',(0.,0.,-1.)) ;
#35032=DIRECTION('',(1.,0.,0.)) ;
#35033=DIRECTION('',(0.,0.,-1.)) ;
#35034=DIRECTION('',(1.,0.,0.)) ;
#35035=DIRECTION('center_axis',(-1.,0.,0.)) ;
#35036=DIRECTION('ref_axis',(0.,0.,1.)) ;
#35037=DIRECTION('',(0.,1.,0.)) ;
#35038=DIRECTION('center_axis',(0.,1.,0.)) ;
#35039=DIRECTION('ref_axis',(0.,0.,1.)) ;
#35040=DIRECTION('',(-1.,0.,0.)) ;
#35041=DIRECTION('center_axis',(0.,1.,0.)) ;
#35042=DIRECTION('ref_axis',(1.,0.,0.)) ;
#35043=DIRECTION('',(1.,0.,0.)) ;
#35044=DIRECTION('',(0.,0.,-1.)) ;
#35045=DIRECTION('center_axis',(0.,1.,0.)) ;
#35046=DIRECTION('ref_axis',(0.,0.,1.)) ;
#35047=DIRECTION('',(0.,0.,-1.)) ;
#35048=DIRECTION('',(1.,0.,0.)) ;
#35049=DIRECTION('center_axis',(0.,1.,0.)) ;
#35050=DIRECTION('ref_axis',(1.,0.,0.)) ;
#35051=DIRECTION('center_axis',(0.,0.,1.)) ;
#35052=DIRECTION('ref_axis',(1.,0.,0.)) ;
#35053=DIRECTION('',(0.,1.,0.)) ;
#35054=DIRECTION('',(-1.,0.,0.)) ;
#35055=DIRECTION('',(0.,1.,0.)) ;
#35056=DIRECTION('center_axis',(0.,0.,1.)) ;
#35057=DIRECTION('ref_axis',(1.,0.,0.)) ;
#35058=DIRECTION('',(-1.,0.,0.)) ;
#35059=DIRECTION('',(0.,1.,0.)) ;
#35060=DIRECTION('',(1.,0.,0.)) ;
#35061=DIRECTION('',(0.,-1.,0.)) ;
#35062=DIRECTION('center_axis',(0.,0.,1.)) ;
#35063=DIRECTION('ref_axis',(1.,0.,0.)) ;
#35064=DIRECTION('',(-1.,0.,0.)) ;
#35065=DIRECTION('',(0.,1.,0.)) ;
#35066=DIRECTION('',(1.,0.,0.)) ;
#35067=DIRECTION('',(0.,-1.,0.)) ;
#35068=DIRECTION('center_axis',(0.,0.,1.)) ;
#35069=DIRECTION('ref_axis',(1.,0.,0.)) ;
#35070=DIRECTION('',(-1.,0.,0.)) ;
#35071=DIRECTION('',(0.,-1.,0.)) ;
#35072=DIRECTION('',(1.,0.,0.)) ;
#35073=DIRECTION('',(0.,1.,0.)) ;
#35074=DIRECTION('center_axis',(0.,0.,1.)) ;
#35075=DIRECTION('ref_axis',(1.,0.,0.)) ;
#35076=DIRECTION('',(0.,-1.,0.)) ;
#35077=DIRECTION('',(-1.,0.,0.)) ;
#35078=DIRECTION('',(0.,-1.,0.)) ;
#35079=DIRECTION('center_axis',(0.,-1.,0.)) ;
#35080=DIRECTION('ref_axis',(0.,0.,-1.)) ;
#35081=DIRECTION('',(0.,0.,-1.)) ;
#35082=DIRECTION('',(-1.,0.,0.)) ;
#35083=DIRECTION('',(0.,0.,-1.)) ;
#35084=DIRECTION('center_axis',(0.,-1.,0.)) ;
#35085=DIRECTION('ref_axis',(1.,0.,0.)) ;
#35086=DIRECTION('center_axis',(0.,-1.,0.)) ;
#35087=DIRECTION('ref_axis',(0.,0.,-1.)) ;
#35088=DIRECTION('',(0.,0.,-1.)) ;
#35089=DIRECTION('',(1.,0.,0.)) ;
#35090=DIRECTION('',(0.,0.,-1.)) ;
#35091=DIRECTION('center_axis',(0.,-1.,0.)) ;
#35092=DIRECTION('ref_axis',(1.,0.,0.)) ;
#35093=DIRECTION('center_axis',(1.,0.,0.)) ;
#35094=DIRECTION('ref_axis',(0.,0.,-1.)) ;
#35095=DIRECTION('',(0.,0.,1.)) ;
#35096=DIRECTION('',(0.,-1.,0.)) ;
#35097=DIRECTION('',(0.,0.,-1.)) ;
#35098=DIRECTION('',(0.,1.,0.)) ;
#35099=DIRECTION('',(0.,0.,1.)) ;
#35100=DIRECTION('',(0.,-1.,0.)) ;
#35101=DIRECTION('',(0.,1.,0.)) ;
#35102=DIRECTION('',(0.,0.,-1.)) ;
#35103=DIRECTION('',(0.,0.,-1.)) ;
#35104=DIRECTION('',(0.,1.,0.)) ;
#35105=DIRECTION('',(0.,0.,-1.)) ;
#35106=DIRECTION('',(0.,0.,-1.)) ;
#35107=DIRECTION('',(0.,-1.,0.)) ;
#35108=DIRECTION('',(0.,0.,-1.)) ;
#35109=DIRECTION('',(0.,1.,0.)) ;
#35110=DIRECTION('',(0.,0.,-1.)) ;
#35111=DIRECTION('',(0.,1.,0.)) ;
#35112=DIRECTION('',(0.,0.,-1.)) ;
#35113=DIRECTION('',(0.,0.,-1.)) ;
#35114=DIRECTION('',(0.,1.,0.)) ;
#35115=DIRECTION('',(0.,0.,-1.)) ;
#35116=DIRECTION('',(0.,-1.,0.)) ;
#35117=DIRECTION('center_axis',(0.,1.,0.)) ;
#35118=DIRECTION('ref_axis',(0.,0.,1.)) ;
#35119=DIRECTION('center_axis',(0.,1.,0.)) ;
#35120=DIRECTION('ref_axis',(1.,0.,0.)) ;
#35121=DIRECTION('',(0.,0.,-1.)) ;
#35122=DIRECTION('',(1.,0.,0.)) ;
#35123=DIRECTION('center_axis',(0.,1.,0.)) ;
#35124=DIRECTION('ref_axis',(0.,0.,1.)) ;
#35125=DIRECTION('',(-1.,0.,0.)) ;
#35126=DIRECTION('',(0.,0.,-1.)) ;
#35127=DIRECTION('center_axis',(0.,-1.,0.)) ;
#35128=DIRECTION('ref_axis',(0.,0.,-1.)) ;
#35129=DIRECTION('',(0.,0.,-1.)) ;
#35130=DIRECTION('',(1.,0.,0.)) ;
#35131=DIRECTION('center_axis',(1.,0.,0.)) ;
#35132=DIRECTION('ref_axis',(0.,0.,-1.)) ;
#35133=DIRECTION('',(0.,0.,-1.)) ;
#35134=DIRECTION('',(0.,-1.,0.)) ;
#35135=DIRECTION('',(0.,0.,-1.)) ;
#35136=DIRECTION('center_axis',(0.,-1.,0.)) ;
#35137=DIRECTION('ref_axis',(0.,0.,-1.)) ;
#35138=DIRECTION('',(-1.,0.,0.)) ;
#35139=DIRECTION('',(0.,0.,-1.)) ;
#35140=DIRECTION('center_axis',(1.,0.,0.)) ;
#35141=DIRECTION('ref_axis',(0.,0.,-1.)) ;
#35142=DIRECTION('',(0.,0.,-1.)) ;
#35143=DIRECTION('',(0.,-1.,0.)) ;
#35144=DIRECTION('',(0.,0.,-1.)) ;
#35145=DIRECTION('center_axis',(0.,-1.,0.)) ;
#35146=DIRECTION('ref_axis',(0.,0.,-1.)) ;
#35147=DIRECTION('',(-1.,0.,0.)) ;
#35148=DIRECTION('',(0.,0.,-1.)) ;
#35149=DIRECTION('center_axis',(0.,0.,1.)) ;
#35150=DIRECTION('ref_axis',(1.,0.,0.)) ;
#35151=DIRECTION('',(0.,-1.,0.)) ;
#35152=DIRECTION('',(1.,0.,0.)) ;
#35153=DIRECTION('',(0.,1.,0.)) ;
#35154=DIRECTION('center_axis',(0.,0.,1.)) ;
#35155=DIRECTION('ref_axis',(1.,0.,0.)) ;
#35156=DIRECTION('',(1.,0.,0.)) ;
#35157=DIRECTION('',(0.,1.,0.)) ;
#35158=DIRECTION('center_axis',(0.,-1.,0.)) ;
#35159=DIRECTION('ref_axis',(0.,0.,-1.)) ;
#35160=DIRECTION('center_axis',(0.,1.,0.)) ;
#35161=DIRECTION('ref_axis',(1.,0.,0.)) ;
#35162=DIRECTION('center_axis',(0.,1.,0.)) ;
#35163=DIRECTION('ref_axis',(0.,0.,1.)) ;
#35164=DIRECTION('center_axis',(0.,-1.,0.)) ;
#35165=DIRECTION('ref_axis',(1.,0.,0.)) ;
#35166=DIRECTION('center_axis',(0.,0.,1.)) ;
#35167=DIRECTION('ref_axis',(1.,0.,0.)) ;
#35168=DIRECTION('',(0.,-1.,0.)) ;
#35169=DIRECTION('',(-1.,0.,0.)) ;
#35170=DIRECTION('',(1.,0.,0.)) ;
#35171=DIRECTION('',(0.,1.,0.)) ;
#35172=DIRECTION('center_axis',(0.,0.,1.)) ;
#35173=DIRECTION('ref_axis',(1.,0.,0.)) ;
#35174=DIRECTION('',(-1.,0.,0.)) ;
#35175=DIRECTION('',(0.,-1.,0.)) ;
#35176=DIRECTION('',(1.,0.,0.)) ;
#35177=DIRECTION('center_axis',(0.,1.,0.)) ;
#35178=DIRECTION('ref_axis',(0.,0.,1.)) ;
#35179=DIRECTION('',(1.,0.,0.)) ;
#35180=DIRECTION('',(0.,0.,-1.)) ;
#35181=DIRECTION('center_axis',(0.,1.,0.)) ;
#35182=DIRECTION('ref_axis',(0.,0.,1.)) ;
#35183=DIRECTION('',(0.,0.,-1.)) ;
#35184=DIRECTION('center_axis',(0.,1.,0.)) ;
#35185=DIRECTION('ref_axis',(1.,0.,0.)) ;
#35186=DIRECTION('center_axis',(0.,1.,0.)) ;
#35187=DIRECTION('ref_axis',(0.,0.,1.)) ;
#35188=DIRECTION('',(0.,0.,-1.)) ;
#35189=DIRECTION('center_axis',(-1.,0.,0.)) ;
#35190=DIRECTION('ref_axis',(0.,0.,1.)) ;
#35191=DIRECTION('center_axis',(0.,1.,0.)) ;
#35192=DIRECTION('ref_axis',(0.,0.,1.)) ;
#35193=DIRECTION('',(0.,0.,-1.)) ;
#35194=DIRECTION('center_axis',(-1.,0.,0.)) ;
#35195=DIRECTION('ref_axis',(0.,0.,1.)) ;
#35196=DIRECTION('center_axis',(0.,1.,0.)) ;
#35197=DIRECTION('ref_axis',(1.,0.,0.)) ;
#35198=DIRECTION('center_axis',(0.,1.,0.)) ;
#35199=DIRECTION('ref_axis',(1.,0.,0.)) ;
#35200=DIRECTION('center_axis',(0.,-1.,0.)) ;
#35201=DIRECTION('ref_axis',(1.,0.,0.)) ;
#35202=DIRECTION('center_axis',(0.,-1.,0.)) ;
#35203=DIRECTION('ref_axis',(-1.,0.,0.)) ;
#35204=DIRECTION('center_axis',(0.,-1.,0.)) ;
#35205=DIRECTION('ref_axis',(1.,0.,0.)) ;
#35206=DIRECTION('center_axis',(0.,1.,0.)) ;
#35207=DIRECTION('ref_axis',(1.,0.,0.)) ;
#35208=DIRECTION('center_axis',(0.,1.,0.)) ;
#35209=DIRECTION('ref_axis',(1.,0.,0.)) ;
#35210=DIRECTION('',(0.,-1.,0.)) ;
#35211=DIRECTION('center_axis',(0.,1.,0.)) ;
#35212=DIRECTION('ref_axis',(1.,0.,0.)) ;
#35213=DIRECTION('',(0.,-1.,0.)) ;
#35214=DIRECTION('center_axis',(0.,1.,0.)) ;
#35215=DIRECTION('ref_axis',(1.,0.,0.)) ;
#35216=DIRECTION('',(0.,1.,0.)) ;
#35217=DIRECTION('center_axis',(0.,1.,0.)) ;
#35218=DIRECTION('ref_axis',(1.,0.,0.)) ;
#35219=DIRECTION('',(0.,1.,0.)) ;
#35220=DIRECTION('center_axis',(0.,0.,1.)) ;
#35221=DIRECTION('ref_axis',(1.,0.,0.)) ;
#35222=DIRECTION('',(1.,0.,0.)) ;
#35223=DIRECTION('',(0.,1.,0.)) ;
#35224=DIRECTION('',(-1.,0.,0.)) ;
#35225=DIRECTION('center_axis',(-1.,0.,0.)) ;
#35226=DIRECTION('ref_axis',(0.,0.,1.)) ;
#35227=DIRECTION('',(0.,0.,-1.)) ;
#35228=DIRECTION('',(0.,-1.,0.)) ;
#35229=DIRECTION('',(0.,0.,-1.)) ;
#35230=DIRECTION('',(0.,1.,0.)) ;
#35231=DIRECTION('center_axis',(1.,0.,0.)) ;
#35232=DIRECTION('ref_axis',(0.,0.,-1.)) ;
#35233=DIRECTION('',(0.,0.,-1.)) ;
#35234=DIRECTION('',(0.,1.,0.)) ;
#35235=DIRECTION('',(0.,0.,-1.)) ;
#35236=DIRECTION('',(0.,-1.,0.)) ;
#35237=DIRECTION('center_axis',(0.,0.,1.)) ;
#35238=DIRECTION('ref_axis',(1.,0.,0.)) ;
#35239=DIRECTION('',(-1.,0.,0.)) ;
#35240=DIRECTION('',(1.,0.,0.)) ;
#35241=DIRECTION('center_axis',(0.,0.,1.)) ;
#35242=DIRECTION('ref_axis',(1.,0.,0.)) ;
#35243=DIRECTION('',(0.,-1.,0.)) ;
#35244=DIRECTION('',(1.,0.,0.)) ;
#35245=DIRECTION('',(-1.,0.,0.)) ;
#35246=DIRECTION('center_axis',(0.,0.,1.)) ;
#35247=DIRECTION('ref_axis',(1.,0.,0.)) ;
#35248=DIRECTION('',(-1.,0.,0.)) ;
#35249=DIRECTION('',(1.,0.,0.)) ;
#35250=DIRECTION('center_axis',(0.,1.,0.)) ;
#35251=DIRECTION('ref_axis',(0.,0.,1.)) ;
#35252=DIRECTION('',(0.,0.,1.)) ;
#35253=DIRECTION('center_axis',(0.,-1.,0.)) ;
#35254=DIRECTION('ref_axis',(0.,0.,-1.)) ;
#35255=DIRECTION('',(0.,0.,-1.)) ;
#35256=DIRECTION('center_axis',(0.,0.,1.)) ;
#35257=DIRECTION('ref_axis',(1.,0.,0.)) ;
#35258=DIRECTION('',(1.,0.,0.)) ;
#35259=DIRECTION('',(0.,-1.,0.)) ;
#35260=DIRECTION('',(-1.,0.,0.)) ;
#35261=DIRECTION('',(0.,1.,0.)) ;
#35262=DIRECTION('center_axis',(0.,0.,1.)) ;
#35263=DIRECTION('ref_axis',(1.,0.,0.)) ;
#35264=DIRECTION('',(0.,-1.,0.)) ;
#35265=DIRECTION('',(0.,-1.,0.)) ;
#35266=DIRECTION('center_axis',(-1.,0.,0.)) ;
#35267=DIRECTION('ref_axis',(0.,0.,1.)) ;
#35268=DIRECTION('',(0.,-1.,0.)) ;
#35269=DIRECTION('center_axis',(1.,0.,0.)) ;
#35270=DIRECTION('ref_axis',(0.,0.,-1.)) ;
#35271=DIRECTION('',(0.,1.,0.)) ;
#35272=DIRECTION('center_axis',(0.,0.,1.)) ;
#35273=DIRECTION('ref_axis',(1.,0.,0.)) ;
#35274=DIRECTION('',(1.,0.,0.)) ;
#35275=DIRECTION('',(0.,1.,0.)) ;
#35276=DIRECTION('',(-1.,0.,0.)) ;
#35277=DIRECTION('',(0.,-1.,0.)) ;
#35278=DIRECTION('center_axis',(1.,0.,0.)) ;
#35279=DIRECTION('ref_axis',(0.,0.,-1.)) ;
#35280=DIRECTION('',(0.,0.,-1.)) ;
#35281=DIRECTION('',(0.,0.,-1.)) ;
#35282=DIRECTION('center_axis',(0.,1.,0.)) ;
#35283=DIRECTION('ref_axis',(0.,0.,1.)) ;
#35284=DIRECTION('',(0.,0.,-1.)) ;
#35285=DIRECTION('center_axis',(-1.,0.,0.)) ;
#35286=DIRECTION('ref_axis',(0.,0.,1.)) ;
#35287=DIRECTION('',(0.,0.,-1.)) ;
#35288=DIRECTION('center_axis',(0.,-1.,0.)) ;
#35289=DIRECTION('ref_axis',(0.,0.,-1.)) ;
#35290=DIRECTION('center_axis',(0.,0.,1.)) ;
#35291=DIRECTION('ref_axis',(1.,0.,0.)) ;
#35292=DIRECTION('center_axis',(0.,0.,1.)) ;
#35293=DIRECTION('ref_axis',(1.,0.,0.)) ;
#35294=DIRECTION('center_axis',(0.,0.,1.)) ;
#35295=DIRECTION('ref_axis',(1.,0.,0.)) ;
#35296=DIRECTION('center_axis',(0.,0.,1.)) ;
#35297=DIRECTION('ref_axis',(1.,0.,0.)) ;
#35298=DIRECTION('center_axis',(0.,0.,-1.)) ;
#35299=DIRECTION('ref_axis',(1.,0.,0.)) ;
#35300=DIRECTION('center_axis',(0.,0.,1.)) ;
#35301=DIRECTION('ref_axis',(1.,0.,0.)) ;
#35302=DIRECTION('',(0.,0.,-1.)) ;
#35303=DIRECTION('center_axis',(0.,0.,-1.)) ;
#35304=DIRECTION('ref_axis',(1.,0.,0.)) ;
#35305=DIRECTION('center_axis',(0.,0.,1.)) ;
#35306=DIRECTION('ref_axis',(1.,0.,0.)) ;
#35307=DIRECTION('',(0.,0.,1.)) ;
#35308=DIRECTION('center_axis',(0.,0.,1.)) ;
#35309=DIRECTION('ref_axis',(1.,0.,0.)) ;
#35310=DIRECTION('center_axis',(0.,0.,-1.)) ;
#35311=DIRECTION('ref_axis',(1.,0.,0.)) ;
#35312=DIRECTION('center_axis',(0.,0.,1.)) ;
#35313=DIRECTION('ref_axis',(1.,0.,0.)) ;
#35314=DIRECTION('center_axis',(0.,0.,1.)) ;
#35315=DIRECTION('ref_axis',(1.,0.,0.)) ;
#35316=DIRECTION('center_axis',(0.,0.,-1.)) ;
#35317=DIRECTION('ref_axis',(1.,0.,0.)) ;
#35318=DIRECTION('center_axis',(0.,0.,1.)) ;
#35319=DIRECTION('ref_axis',(1.,0.,0.)) ;
#35320=DIRECTION('',(0.,0.,-1.)) ;
#35321=DIRECTION('center_axis',(0.,0.,1.)) ;
#35322=DIRECTION('ref_axis',(1.,0.,0.)) ;
#35323=DIRECTION('',(0.,0.,1.)) ;
#35324=DIRECTION('center_axis',(0.,1.,0.)) ;
#35325=DIRECTION('ref_axis',(1.,0.,0.)) ;
#35326=DIRECTION('',(0.,1.,0.)) ;
#35327=DIRECTION('center_axis',(0.,1.,0.)) ;
#35328=DIRECTION('ref_axis',(1.,0.,0.)) ;
#35329=DIRECTION('center_axis',(0.,-1.,0.)) ;
#35330=DIRECTION('ref_axis',(1.,0.,0.)) ;
#35331=DIRECTION('center_axis',(0.,-1.,0.)) ;
#35332=DIRECTION('ref_axis',(1.,0.,0.)) ;
#35333=DIRECTION('center_axis',(0.,-1.,0.)) ;
#35334=DIRECTION('ref_axis',(0.,0.,-1.)) ;
#35335=DIRECTION('',(1.,0.,0.)) ;
#35336=DIRECTION('center_axis',(0.,-1.,0.)) ;
#35337=DIRECTION('ref_axis',(0.,0.,-1.)) ;
#35338=DIRECTION('',(0.,0.,-1.)) ;
#35339=DIRECTION('center_axis',(0.,-1.,0.)) ;
#35340=DIRECTION('ref_axis',(0.,0.,-1.)) ;
#35341=DIRECTION('',(0.,0.,-1.)) ;
#35342=DIRECTION('center_axis',(-1.,0.,0.)) ;
#35343=DIRECTION('ref_axis',(0.,0.,1.)) ;
#35344=DIRECTION('',(0.,0.,-1.)) ;
#35345=DIRECTION('',(0.,-1.,0.)) ;
#35346=DIRECTION('',(0.,0.,-1.)) ;
#35347=DIRECTION('center_axis',(0.,-1.,0.)) ;
#35348=DIRECTION('ref_axis',(0.,0.,-1.)) ;
#35349=DIRECTION('',(1.,0.,0.)) ;
#35350=DIRECTION('',(1.,0.,0.)) ;
#35351=DIRECTION('center_axis',(0.,0.,1.)) ;
#35352=DIRECTION('ref_axis',(1.,0.,0.)) ;
#35353=DIRECTION('center_axis',(0.,0.,1.)) ;
#35354=DIRECTION('ref_axis',(1.,0.,0.)) ;
#35355=DIRECTION('center_axis',(0.,0.,1.)) ;
#35356=DIRECTION('ref_axis',(1.,0.,0.)) ;
#35357=DIRECTION('',(-1.,0.,0.)) ;
#35358=DIRECTION('center_axis',(0.,1.,0.)) ;
#35359=DIRECTION('ref_axis',(0.,0.,1.)) ;
#35360=DIRECTION('',(0.,0.,-1.)) ;
#35361=DIRECTION('center_axis',(0.,0.,1.)) ;
#35362=DIRECTION('ref_axis',(1.,0.,0.)) ;
#35363=DIRECTION('',(-1.,0.,0.)) ;
#35364=DIRECTION('',(0.,1.,0.)) ;
#35365=DIRECTION('center_axis',(-1.,0.,0.)) ;
#35366=DIRECTION('ref_axis',(0.,0.,1.)) ;
#35367=DIRECTION('',(0.,0.,-1.)) ;
#35368=DIRECTION('',(0.,-1.,0.)) ;
#35369=DIRECTION('',(0.,0.,1.)) ;
#35370=DIRECTION('center_axis',(-1.,0.,0.)) ;
#35371=DIRECTION('ref_axis',(0.,0.,1.)) ;
#35372=DIRECTION('',(0.,0.,-1.)) ;
#35373=DIRECTION('',(0.,-1.,0.)) ;
#35374=DIRECTION('',(0.,0.,-1.)) ;
#35375=DIRECTION('',(0.,1.,0.)) ;
#35376=DIRECTION('center_axis',(1.,0.,0.)) ;
#35377=DIRECTION('ref_axis',(0.,0.,-1.)) ;
#35378=DIRECTION('',(0.,0.,-1.)) ;
#35379=DIRECTION('',(0.,1.,0.)) ;
#35380=DIRECTION('',(0.,0.,-1.)) ;
#35381=DIRECTION('',(0.,-1.,0.)) ;
#35382=DIRECTION('center_axis',(0.,1.,0.)) ;
#35383=DIRECTION('ref_axis',(0.,0.,1.)) ;
#35384=DIRECTION('',(-1.,0.,0.)) ;
#35385=DIRECTION('',(1.,0.,0.)) ;
#35386=DIRECTION('',(-1.,0.,0.)) ;
#35387=DIRECTION('center_axis',(0.,0.,1.)) ;
#35388=DIRECTION('ref_axis',(1.,0.,0.)) ;
#35389=DIRECTION('',(1.,0.,0.)) ;
#35390=DIRECTION('center_axis',(0.,0.,1.)) ;
#35391=DIRECTION('ref_axis',(1.,0.,0.)) ;
#35392=DIRECTION('',(-1.,0.,0.)) ;
#35393=DIRECTION('center_axis',(0.,-1.,0.)) ;
#35394=DIRECTION('ref_axis',(0.,0.,-1.)) ;
#35395=DIRECTION('',(1.,0.,0.)) ;
#35396=DIRECTION('center_axis',(0.,0.,1.)) ;
#35397=DIRECTION('ref_axis',(1.,0.,0.)) ;
#35398=DIRECTION('center_axis',(0.,1.,0.)) ;
#35399=DIRECTION('ref_axis',(1.,0.,0.)) ;
#35400=DIRECTION('center_axis',(0.,-1.,0.)) ;
#35401=DIRECTION('ref_axis',(1.,0.,0.)) ;
#35402=DIRECTION('',(0.,-1.,0.)) ;
#35403=DIRECTION('center_axis',(0.,1.,0.)) ;
#35404=DIRECTION('ref_axis',(1.,0.,0.)) ;
#35405=DIRECTION('',(0.,1.,0.)) ;
#35406=DIRECTION('center_axis',(1.,0.,0.)) ;
#35407=DIRECTION('ref_axis',(0.,0.,-1.)) ;
#35408=DIRECTION('',(0.,0.,-1.)) ;
#35409=DIRECTION('',(0.,-1.,0.)) ;
#35410=DIRECTION('',(0.,0.,-1.)) ;
#35411=DIRECTION('center_axis',(0.,-1.,0.)) ;
#35412=DIRECTION('ref_axis',(0.,0.,-1.)) ;
#35413=DIRECTION('',(0.,0.,-1.)) ;
#35414=DIRECTION('',(-1.,0.,0.)) ;
#35415=DIRECTION('center_axis',(-1.,0.,0.)) ;
#35416=DIRECTION('ref_axis',(0.,0.,1.)) ;
#35417=DIRECTION('',(0.,0.,-1.)) ;
#35418=DIRECTION('',(0.,1.,0.)) ;
#35419=DIRECTION('center_axis',(0.,1.,0.)) ;
#35420=DIRECTION('ref_axis',(0.,0.,1.)) ;
#35421=DIRECTION('',(1.,0.,0.)) ;
#35422=DIRECTION('center_axis',(0.,0.,1.)) ;
#35423=DIRECTION('ref_axis',(1.,0.,0.)) ;
#35424=DIRECTION('center_axis',(0.,0.,1.)) ;
#35425=DIRECTION('ref_axis',(1.,0.,0.)) ;
#35426=DIRECTION('',(-1.,0.,0.)) ;
#35427=DIRECTION('',(0.,1.,0.)) ;
#35428=DIRECTION('',(1.,0.,0.)) ;
#35429=DIRECTION('',(0.,-1.,0.)) ;
#35430=DIRECTION('center_axis',(0.,1.,0.)) ;
#35431=DIRECTION('ref_axis',(0.,0.,1.)) ;
#35432=DIRECTION('center_axis',(0.,-1.,0.)) ;
#35433=DIRECTION('ref_axis',(1.,0.,0.)) ;
#35434=DIRECTION('',(0.,0.,-1.)) ;
#35435=DIRECTION('',(0.,0.,-1.)) ;
#35436=DIRECTION('center_axis',(-1.,0.,0.)) ;
#35437=DIRECTION('ref_axis',(0.,0.,1.)) ;
#35438=DIRECTION('',(0.,-1.,0.)) ;
#35439=DIRECTION('',(0.,0.,-1.)) ;
#35440=DIRECTION('center_axis',(0.,-1.,0.)) ;
#35441=DIRECTION('ref_axis',(0.,0.,-1.)) ;
#35442=DIRECTION('center_axis',(0.,1.,0.)) ;
#35443=DIRECTION('ref_axis',(1.,0.,0.)) ;
#35444=DIRECTION('',(0.,0.,-1.)) ;
#35445=DIRECTION('center_axis',(1.,0.,0.)) ;
#35446=DIRECTION('ref_axis',(0.,0.,-1.)) ;
#35447=DIRECTION('',(0.,1.,0.)) ;
#35448=DIRECTION('center_axis',(0.,1.,0.)) ;
#35449=DIRECTION('ref_axis',(1.,0.,0.)) ;
#35450=DIRECTION('center_axis',(0.,-1.,0.)) ;
#35451=DIRECTION('ref_axis',(0.,0.,-1.)) ;
#35452=DIRECTION('center_axis',(0.,1.,0.)) ;
#35453=DIRECTION('ref_axis',(1.,0.,0.)) ;
#35454=DIRECTION('',(1.,0.,0.)) ;
#35455=DIRECTION('center_axis',(0.,1.,0.)) ;
#35456=DIRECTION('ref_axis',(0.,0.,1.)) ;
#35457=DIRECTION('center_axis',(0.,-1.,0.)) ;
#35458=DIRECTION('ref_axis',(1.,0.,0.)) ;
#35459=DIRECTION('',(-1.,0.,0.)) ;
#35460=DIRECTION('center_axis',(0.,0.,1.)) ;
#35461=DIRECTION('ref_axis',(1.,0.,0.)) ;
#35462=DIRECTION('',(0.,-1.,0.)) ;
#35463=DIRECTION('',(0.,1.,0.)) ;
#35464=DIRECTION('center_axis',(0.,1.,0.)) ;
#35465=DIRECTION('ref_axis',(1.,0.,0.)) ;
#35466=DIRECTION('center_axis',(0.,0.,1.)) ;
#35467=DIRECTION('ref_axis',(1.,0.,0.)) ;
#35468=DIRECTION('',(1.,0.,0.)) ;
#35469=DIRECTION('',(0.,1.,0.)) ;
#35470=DIRECTION('',(-1.,0.,0.)) ;
#35471=DIRECTION('',(0.,-1.,0.)) ;
#35472=DIRECTION('center_axis',(-1.,0.,0.)) ;
#35473=DIRECTION('ref_axis',(0.,0.,1.)) ;
#35474=DIRECTION('',(0.,0.,1.)) ;
#35475=DIRECTION('',(0.,0.,-1.)) ;
#35476=DIRECTION('',(0.,-1.,0.)) ;
#35477=DIRECTION('center_axis',(0.,1.,0.)) ;
#35478=DIRECTION('ref_axis',(0.,0.,1.)) ;
#35479=DIRECTION('center_axis',(0.,1.,0.)) ;
#35480=DIRECTION('ref_axis',(1.,0.,0.)) ;
#35481=DIRECTION('center_axis',(0.,-1.,0.)) ;
#35482=DIRECTION('ref_axis',(0.,0.,-1.)) ;
#35483=DIRECTION('center_axis',(0.,-1.,0.)) ;
#35484=DIRECTION('ref_axis',(1.,0.,0.)) ;
#35485=DIRECTION('center_axis',(0.,1.,0.)) ;
#35486=DIRECTION('ref_axis',(1.,0.,0.)) ;
#35487=DIRECTION('center_axis',(0.,-1.,0.)) ;
#35488=DIRECTION('ref_axis',(0.,0.,-1.)) ;
#35489=DIRECTION('',(1.,0.,0.)) ;
#35490=DIRECTION('center_axis',(0.,1.,0.)) ;
#35491=DIRECTION('ref_axis',(1.,0.,0.)) ;
#35492=DIRECTION('',(0.,0.,-1.)) ;
#35493=DIRECTION('center_axis',(1.,0.,0.)) ;
#35494=DIRECTION('ref_axis',(0.,0.,-1.)) ;
#35495=DIRECTION('',(0.,1.,0.)) ;
#35496=DIRECTION('',(0.,-1.,0.)) ;
#35497=DIRECTION('',(0.,0.,-1.)) ;
#35498=DIRECTION('center_axis',(0.,1.,0.)) ;
#35499=DIRECTION('ref_axis',(0.,0.,1.)) ;
#35500=DIRECTION('',(-1.,0.,0.)) ;
#35501=DIRECTION('center_axis',(0.,-1.,0.)) ;
#35502=DIRECTION('ref_axis',(1.,0.,0.)) ;
#35503=DIRECTION('center_axis',(0.,1.,0.)) ;
#35504=DIRECTION('ref_axis',(1.,0.,0.)) ;
#35505=DIRECTION('',(0.,-1.,0.)) ;
#35506=DIRECTION('center_axis',(0.,0.,1.)) ;
#35507=DIRECTION('ref_axis',(1.,0.,0.)) ;
#35508=DIRECTION('center_axis',(0.,0.,1.)) ;
#35509=DIRECTION('ref_axis',(1.,0.,0.)) ;
#35510=DIRECTION('',(1.,0.,0.)) ;
#35511=DIRECTION('',(0.,1.,0.)) ;
#35512=DIRECTION('',(-1.,0.,0.)) ;
#35513=DIRECTION('',(0.,-1.,0.)) ;
#35514=DIRECTION('center_axis',(1.,0.,0.)) ;
#35515=DIRECTION('ref_axis',(0.,0.,-1.)) ;
#35516=DIRECTION('',(0.,0.,-1.)) ;
#35517=DIRECTION('',(0.,1.,0.)) ;
#35518=DIRECTION('',(0.,0.,1.)) ;
#35519=DIRECTION('center_axis',(0.,1.,0.)) ;
#35520=DIRECTION('ref_axis',(0.,0.,1.)) ;
#35521=DIRECTION('center_axis',(0.,1.,0.)) ;
#35522=DIRECTION('ref_axis',(1.,0.,0.)) ;
#35523=DIRECTION('center_axis',(0.,-1.,0.)) ;
#35524=DIRECTION('ref_axis',(0.,0.,-1.)) ;
#35525=DIRECTION('center_axis',(0.,-1.,0.)) ;
#35526=DIRECTION('ref_axis',(1.,0.,0.)) ;
#35527=DIRECTION('center_axis',(0.,1.,0.)) ;
#35528=DIRECTION('ref_axis',(1.,0.,0.)) ;
#35529=DIRECTION('center_axis',(0.,-1.,0.)) ;
#35530=DIRECTION('ref_axis',(0.,0.,-1.)) ;
#35531=DIRECTION('',(1.,0.,0.)) ;
#35532=DIRECTION('',(0.,0.,-1.)) ;
#35533=DIRECTION('center_axis',(0.,1.,0.)) ;
#35534=DIRECTION('ref_axis',(1.,0.,0.)) ;
#35535=DIRECTION('center_axis',(0.,1.,0.)) ;
#35536=DIRECTION('ref_axis',(0.,0.,1.)) ;
#35537=DIRECTION('',(-1.,0.,0.)) ;
#35538=DIRECTION('center_axis',(0.,-1.,0.)) ;
#35539=DIRECTION('ref_axis',(1.,0.,0.)) ;
#35540=DIRECTION('',(0.,0.,-1.)) ;
#35541=DIRECTION('center_axis',(0.,1.,0.)) ;
#35542=DIRECTION('ref_axis',(1.,0.,0.)) ;
#35543=DIRECTION('',(0.,1.,0.)) ;
#35544=DIRECTION('',(0.,1.,0.)) ;
#35545=DIRECTION('center_axis',(-1.,0.,0.)) ;
#35546=DIRECTION('ref_axis',(0.,0.,1.)) ;
#35547=DIRECTION('',(0.,-1.,0.)) ;
#35548=DIRECTION('center_axis',(0.,0.,1.)) ;
#35549=DIRECTION('ref_axis',(1.,0.,0.)) ;
#35550=DIRECTION('center_axis',(0.,0.,1.)) ;
#35551=DIRECTION('ref_axis',(1.,0.,0.)) ;
#35552=DIRECTION('',(-1.,0.,0.)) ;
#35553=DIRECTION('',(0.,-1.,0.)) ;
#35554=DIRECTION('',(1.,0.,0.)) ;
#35555=DIRECTION('',(0.,1.,0.)) ;
#35556=DIRECTION('center_axis',(0.,1.,0.)) ;
#35557=DIRECTION('ref_axis',(1.,0.,0.)) ;
#35558=DIRECTION('center_axis',(0.,-1.,0.)) ;
#35559=DIRECTION('ref_axis',(1.,0.,0.)) ;
#35560=DIRECTION('',(0.,-1.,0.)) ;
#35561=DIRECTION('center_axis',(0.,1.,0.)) ;
#35562=DIRECTION('ref_axis',(1.,0.,0.)) ;
#35563=DIRECTION('center_axis',(0.,1.,0.)) ;
#35564=DIRECTION('ref_axis',(0.,0.,1.)) ;
#35565=DIRECTION('',(0.,0.,-1.)) ;
#35566=DIRECTION('center_axis',(1.,0.,0.)) ;
#35567=DIRECTION('ref_axis',(0.,0.,-1.)) ;
#35568=DIRECTION('',(0.,0.,-1.)) ;
#35569=DIRECTION('center_axis',(0.,-1.,0.)) ;
#35570=DIRECTION('ref_axis',(0.,0.,-1.)) ;
#35571=DIRECTION('center_axis',(0.,-1.,0.)) ;
#35572=DIRECTION('ref_axis',(0.,0.,-1.)) ;
#35573=DIRECTION('',(1.,0.,0.)) ;
#35574=DIRECTION('',(0.,0.,-1.)) ;
#35575=DIRECTION('center_axis',(0.,1.,0.)) ;
#35576=DIRECTION('ref_axis',(1.,0.,0.)) ;
#35577=DIRECTION('center_axis',(0.,1.,0.)) ;
#35578=DIRECTION('ref_axis',(0.,0.,1.)) ;
#35579=DIRECTION('',(-1.,0.,0.)) ;
#35580=DIRECTION('center_axis',(0.,-1.,0.)) ;
#35581=DIRECTION('ref_axis',(1.,0.,0.)) ;
#35582=DIRECTION('',(0.,0.,-1.)) ;
#35583=DIRECTION('center_axis',(0.,1.,0.)) ;
#35584=DIRECTION('ref_axis',(1.,0.,0.)) ;
#35585=DIRECTION('',(0.,1.,0.)) ;
#35586=DIRECTION('',(0.,1.,0.)) ;
#35587=DIRECTION('center_axis',(-1.,0.,0.)) ;
#35588=DIRECTION('ref_axis',(0.,0.,1.)) ;
#35589=DIRECTION('',(0.,-1.,0.)) ;
#35590=DIRECTION('center_axis',(0.,0.,1.)) ;
#35591=DIRECTION('ref_axis',(1.,0.,0.)) ;
#35592=DIRECTION('center_axis',(0.,0.,1.)) ;
#35593=DIRECTION('ref_axis',(1.,0.,0.)) ;
#35594=DIRECTION('',(0.,-1.,0.)) ;
#35595=DIRECTION('',(-1.,0.,0.)) ;
#35596=DIRECTION('',(0.,1.,0.)) ;
#35597=DIRECTION('',(1.,0.,0.)) ;
#35598=DIRECTION('center_axis',(0.,1.,0.)) ;
#35599=DIRECTION('ref_axis',(0.,0.,1.)) ;
#35600=DIRECTION('center_axis',(0.,1.,0.)) ;
#35601=DIRECTION('ref_axis',(1.,0.,0.)) ;
#35602=DIRECTION('center_axis',(0.,-1.,0.)) ;
#35603=DIRECTION('ref_axis',(0.,0.,-1.)) ;
#35604=DIRECTION('center_axis',(0.,-1.,0.)) ;
#35605=DIRECTION('ref_axis',(1.,0.,0.)) ;
#35606=DIRECTION('center_axis',(0.,1.,0.)) ;
#35607=DIRECTION('ref_axis',(6.12323399573677E-17,0.,-1.)) ;
#35608=DIRECTION('center_axis',(0.,1.,0.)) ;
#35609=DIRECTION('ref_axis',(6.12323399573677E-17,0.,-1.)) ;
#35610=DIRECTION('',(0.,1.,0.)) ;
#35611=DIRECTION('center_axis',(0.,-1.,0.)) ;
#35612=DIRECTION('ref_axis',(1.,0.,0.)) ;
#35613=DIRECTION('',(0.,-1.,0.)) ;
#35614=DIRECTION('center_axis',(0.,1.,0.)) ;
#35615=DIRECTION('ref_axis',(1.,0.,0.)) ;
#35616=DIRECTION('center_axis',(0.,1.,0.)) ;
#35617=DIRECTION('ref_axis',(0.,0.,1.)) ;
#35618=DIRECTION('',(1.,0.,0.)) ;
#35619=DIRECTION('center_axis',(0.,-1.,0.)) ;
#35620=DIRECTION('ref_axis',(0.,0.,-1.)) ;
#35621=DIRECTION('',(-1.,0.,0.)) ;
#35622=DIRECTION('center_axis',(0.,0.,1.)) ;
#35623=DIRECTION('ref_axis',(1.,0.,0.)) ;
#35624=DIRECTION('center_axis',(0.,0.,1.)) ;
#35625=DIRECTION('ref_axis',(1.,0.,0.)) ;
#35626=DIRECTION('',(-1.,0.,0.)) ;
#35627=DIRECTION('',(0.,-1.,0.)) ;
#35628=DIRECTION('',(1.,0.,0.)) ;
#35629=DIRECTION('',(0.,1.,0.)) ;
#35630=DIRECTION('center_axis',(0.,-1.,0.)) ;
#35631=DIRECTION('ref_axis',(0.,0.,-1.)) ;
#35632=DIRECTION('center_axis',(0.,-1.,0.)) ;
#35633=DIRECTION('ref_axis',(1.,0.,0.)) ;
#35634=DIRECTION('center_axis',(0.,1.,0.)) ;
#35635=DIRECTION('ref_axis',(0.,0.,1.)) ;
#35636=DIRECTION('center_axis',(0.,1.,0.)) ;
#35637=DIRECTION('ref_axis',(1.,0.,0.)) ;
#35638=DIRECTION('center_axis',(0.,1.,0.)) ;
#35639=DIRECTION('ref_axis',(1.,0.,0.)) ;
#35640=DIRECTION('center_axis',(0.,1.,0.)) ;
#35641=DIRECTION('ref_axis',(6.12323399573677E-17,0.,-1.)) ;
#35642=DIRECTION('',(0.,1.,0.)) ;
#35643=DIRECTION('center_axis',(0.,-1.,0.)) ;
#35644=DIRECTION('ref_axis',(1.,0.,0.)) ;
#35645=DIRECTION('',(0.,-1.,0.)) ;
#35646=DIRECTION('center_axis',(0.,1.,0.)) ;
#35647=DIRECTION('ref_axis',(1.,0.,0.)) ;
#35648=DIRECTION('center_axis',(0.,1.,0.)) ;
#35649=DIRECTION('ref_axis',(0.,0.,1.)) ;
#35650=DIRECTION('',(-1.,0.,0.)) ;
#35651=DIRECTION('center_axis',(0.,-1.,0.)) ;
#35652=DIRECTION('ref_axis',(0.,0.,-1.)) ;
#35653=DIRECTION('',(1.,0.,0.)) ;
#35654=DIRECTION('center_axis',(0.,0.,1.)) ;
#35655=DIRECTION('ref_axis',(1.,0.,0.)) ;
#35656=DIRECTION('center_axis',(0.,0.,1.)) ;
#35657=DIRECTION('ref_axis',(1.,0.,0.)) ;
#35658=DIRECTION('',(0.,1.,0.)) ;
#35659=DIRECTION('',(-1.,0.,0.)) ;
#35660=DIRECTION('',(0.,-1.,0.)) ;
#35661=DIRECTION('',(1.,0.,0.)) ;
#35662=DIRECTION('center_axis',(0.,1.,0.)) ;
#35663=DIRECTION('ref_axis',(0.,0.,1.)) ;
#35664=DIRECTION('center_axis',(0.,1.,0.)) ;
#35665=DIRECTION('ref_axis',(1.,0.,0.)) ;
#35666=DIRECTION('center_axis',(0.,1.,0.)) ;
#35667=DIRECTION('ref_axis',(1.,0.,0.)) ;
#35668=DIRECTION('center_axis',(0.,-1.,0.)) ;
#35669=DIRECTION('ref_axis',(1.,0.,0.)) ;
#35670=DIRECTION('center_axis',(0.,-1.,0.)) ;
#35671=DIRECTION('ref_axis',(0.,0.,-1.)) ;
#35672=DIRECTION('center_axis',(0.,-1.,0.)) ;
#35673=DIRECTION('ref_axis',(0.,0.,-1.)) ;
#35674=DIRECTION('',(-1.,0.,0.)) ;
#35675=DIRECTION('',(0.,0.,-1.)) ;
#35676=DIRECTION('',(1.,0.,0.)) ;
#35677=DIRECTION('',(0.,0.,-1.)) ;
#35678=DIRECTION('center_axis',(1.,0.,0.)) ;
#35679=DIRECTION('ref_axis',(0.,0.,-1.)) ;
#35680=DIRECTION('',(0.,-1.,0.)) ;
#35681=DIRECTION('',(0.,0.,-1.)) ;
#35682=DIRECTION('',(0.,1.,0.)) ;
#35683=DIRECTION('center_axis',(-1.,0.,0.)) ;
#35684=DIRECTION('ref_axis',(0.,0.,1.)) ;
#35685=DIRECTION('',(0.,1.,0.)) ;
#35686=DIRECTION('',(0.,-1.,0.)) ;
#35687=DIRECTION('',(0.,0.,-1.)) ;
#35688=DIRECTION('center_axis',(0.,1.,0.)) ;
#35689=DIRECTION('ref_axis',(0.,0.,1.)) ;
#35690=DIRECTION('',(1.,0.,0.)) ;
#35691=DIRECTION('',(-1.,0.,0.)) ;
#35692=DIRECTION('center_axis',(0.,0.,1.)) ;
#35693=DIRECTION('ref_axis',(1.,0.,0.)) ;
#35694=DIRECTION('center_axis',(0.,0.,1.)) ;
#35695=DIRECTION('ref_axis',(1.,0.,0.)) ;
#35696=DIRECTION('center_axis',(0.,0.,1.)) ;
#35697=DIRECTION('ref_axis',(1.,0.,0.)) ;
#35698=DIRECTION('',(1.,0.,0.)) ;
#35699=DIRECTION('',(0.,-1.,0.)) ;
#35700=DIRECTION('',(-1.,0.,0.)) ;
#35701=DIRECTION('',(0.,1.,0.)) ;
#35702=DIRECTION('center_axis',(0.,0.,1.)) ;
#35703=DIRECTION('ref_axis',(1.,0.,0.)) ;
#35704=DIRECTION('',(-1.,0.,0.)) ;
#35705=DIRECTION('',(0.,-1.,0.)) ;
#35706=DIRECTION('',(1.,0.,0.)) ;
#35707=DIRECTION('',(0.,1.,0.)) ;
#35708=DIRECTION('center_axis',(0.,1.,0.)) ;
#35709=DIRECTION('ref_axis',(0.,0.,1.)) ;
#35710=DIRECTION('',(0.,0.,-1.)) ;
#35711=DIRECTION('',(0.,0.,-1.)) ;
#35712=DIRECTION('center_axis',(-1.,0.,0.)) ;
#35713=DIRECTION('ref_axis',(0.,0.,1.)) ;
#35714=DIRECTION('',(0.,0.,-1.)) ;
#35715=DIRECTION('center_axis',(1.,0.,0.)) ;
#35716=DIRECTION('ref_axis',(0.,0.,-1.)) ;
#35717=DIRECTION('',(0.,0.,-1.)) ;
#35718=DIRECTION('center_axis',(0.,-1.,0.)) ;
#35719=DIRECTION('ref_axis',(0.,0.,-1.)) ;
#35720=DIRECTION('center_axis',(0.,1.,0.)) ;
#35721=DIRECTION('ref_axis',(0.,0.,1.)) ;
#35722=DIRECTION('',(0.,0.,1.)) ;
#35723=DIRECTION('',(-1.,0.,0.)) ;
#35724=DIRECTION('',(0.,0.,-1.)) ;
#35725=DIRECTION('',(1.,0.,0.)) ;
#35726=DIRECTION('center_axis',(0.,0.,1.)) ;
#35727=DIRECTION('ref_axis',(1.,0.,0.)) ;
#35728=DIRECTION('',(0.,-1.,0.)) ;
#35729=DIRECTION('',(1.,0.,0.)) ;
#35730=DIRECTION('',(0.,1.,0.)) ;
#35731=DIRECTION('center_axis',(0.,-1.,0.)) ;
#35732=DIRECTION('ref_axis',(0.,0.,-1.)) ;
#35733=DIRECTION('',(0.,0.,-1.)) ;
#35734=DIRECTION('',(-1.,0.,0.)) ;
#35735=DIRECTION('',(0.,0.,1.)) ;
#35736=DIRECTION('center_axis',(-1.,0.,0.)) ;
#35737=DIRECTION('ref_axis',(0.,0.,1.)) ;
#35738=DIRECTION('',(0.,1.,0.)) ;
#35739=DIRECTION('',(0.,0.,-1.)) ;
#35740=DIRECTION('',(0.,1.,0.)) ;
#35741=DIRECTION('',(0.,0.,1.)) ;
#35742=DIRECTION('',(0.,1.,0.)) ;
#35743=DIRECTION('',(0.,0.,1.)) ;
#35744=DIRECTION('',(0.,-1.,0.)) ;
#35745=DIRECTION('',(0.,0.,-1.)) ;
#35746=DIRECTION('',(0.,1.,0.)) ;
#35747=DIRECTION('center_axis',(0.,0.,1.)) ;
#35748=DIRECTION('ref_axis',(1.,0.,0.)) ;
#35749=DIRECTION('',(0.,-1.,0.)) ;
#35750=DIRECTION('',(1.,0.,0.)) ;
#35751=DIRECTION('center_axis',(0.,0.,1.)) ;
#35752=DIRECTION('ref_axis',(1.,0.,0.)) ;
#35753=DIRECTION('',(1.,0.,0.)) ;
#35754=DIRECTION('',(0.,-1.,0.)) ;
#35755=DIRECTION('center_axis',(1.,0.,0.)) ;
#35756=DIRECTION('ref_axis',(0.,0.,-1.)) ;
#35757=DIRECTION('',(0.,0.,1.)) ;
#35758=DIRECTION('',(0.,1.,0.)) ;
#35759=DIRECTION('',(0.,0.,-1.)) ;
#35760=DIRECTION('',(0.,-1.,0.)) ;
#35761=DIRECTION('',(0.,0.,-1.)) ;
#35762=DIRECTION('',(0.,-1.,0.)) ;
#35763=DIRECTION('',(0.,0.,1.)) ;
#35764=DIRECTION('center_axis',(0.,0.,1.)) ;
#35765=DIRECTION('ref_axis',(1.,0.,0.)) ;
#35766=DIRECTION('',(1.,0.,0.)) ;
#35767=DIRECTION('',(-1.,0.,0.)) ;
#35768=DIRECTION('center_axis',(0.,-1.,0.)) ;
#35769=DIRECTION('ref_axis',(0.,0.,-1.)) ;
#35770=DIRECTION('center_axis',(0.,1.,0.)) ;
#35771=DIRECTION('ref_axis',(0.,0.,1.)) ;
#35772=DIRECTION('',(-1.,0.,0.)) ;
#35773=DIRECTION('center_axis',(0.,0.,1.)) ;
#35774=DIRECTION('ref_axis',(1.,0.,0.)) ;
#35775=DIRECTION('',(-1.,0.,0.)) ;
#35776=DIRECTION('center_axis',(0.,-1.,0.)) ;
#35777=DIRECTION('ref_axis',(0.,0.,-1.)) ;
#35778=DIRECTION('',(1.,0.,0.)) ;
#35779=DIRECTION('center_axis',(0.,0.,1.)) ;
#35780=DIRECTION('ref_axis',(1.,0.,0.)) ;
#35781=DIRECTION('',(-1.,0.,0.)) ;
#35782=DIRECTION('center_axis',(0.,1.,0.)) ;
#35783=DIRECTION('ref_axis',(0.,0.,1.)) ;
#35784=DIRECTION('center_axis',(0.,1.,0.)) ;
#35785=DIRECTION('ref_axis',(1.,0.,0.)) ;
#35786=DIRECTION('',(0.,1.,0.)) ;
#35787=DIRECTION('center_axis',(0.,1.,0.)) ;
#35788=DIRECTION('ref_axis',(1.,0.,0.)) ;
#35789=DIRECTION('',(0.,-1.,0.)) ;
#35790=DIRECTION('center_axis',(0.,-1.,0.)) ;
#35791=DIRECTION('ref_axis',(1.,0.,0.)) ;
#35792=DIRECTION('center_axis',(0.,0.,1.)) ;
#35793=DIRECTION('ref_axis',(1.,0.,0.)) ;
#35794=DIRECTION('',(1.,0.,0.)) ;
#35795=DIRECTION('',(-1.,0.,0.)) ;
#35796=DIRECTION('center_axis',(0.,1.,0.)) ;
#35797=DIRECTION('ref_axis',(0.,0.,1.)) ;
#35798=DIRECTION('center_axis',(0.,-1.,0.)) ;
#35799=DIRECTION('ref_axis',(0.,0.,-1.)) ;
#35800=DIRECTION('center_axis',(0.,-1.,0.)) ;
#35801=DIRECTION('ref_axis',(0.,0.,-1.)) ;
#35802=DIRECTION('center_axis',(0.,-1.,0.)) ;
#35803=DIRECTION('ref_axis',(1.,0.,0.)) ;
#35804=DIRECTION('',(1.,0.,0.)) ;
#35805=DIRECTION('center_axis',(0.,0.,1.)) ;
#35806=DIRECTION('ref_axis',(1.,0.,0.)) ;
#35807=DIRECTION('',(0.,1.,0.)) ;
#35808=DIRECTION('',(1.,0.,0.)) ;
#35809=DIRECTION('',(0.,-1.,0.)) ;
#35810=DIRECTION('center_axis',(0.,1.,0.)) ;
#35811=DIRECTION('ref_axis',(1.,0.,0.)) ;
#35812=DIRECTION('center_axis',(0.,1.,0.)) ;
#35813=DIRECTION('ref_axis',(1.,0.,0.)) ;
#35814=DIRECTION('',(0.,1.,0.)) ;
#35815=DIRECTION('center_axis',(0.,-1.,0.)) ;
#35816=DIRECTION('ref_axis',(1.,0.,0.)) ;
#35817=DIRECTION('',(0.,-1.,0.)) ;
#35818=DIRECTION('center_axis',(0.,1.,0.)) ;
#35819=DIRECTION('ref_axis',(1.,0.,0.)) ;
#35820=DIRECTION('',(0.,1.,0.)) ;
#35821=DIRECTION('center_axis',(0.,-1.,0.)) ;
#35822=DIRECTION('ref_axis',(1.,0.,0.)) ;
#35823=DIRECTION('',(0.,-1.,0.)) ;
#35824=DIRECTION('center_axis',(0.,1.,0.)) ;
#35825=DIRECTION('ref_axis',(1.,0.,0.)) ;
#35826=DIRECTION('center_axis',(0.,1.,0.)) ;
#35827=DIRECTION('ref_axis',(0.,0.,1.)) ;
#35828=DIRECTION('',(-1.,0.,0.)) ;
#35829=DIRECTION('center_axis',(0.,0.,1.)) ;
#35830=DIRECTION('ref_axis',(1.,0.,0.)) ;
#35831=DIRECTION('',(-1.,0.,0.)) ;
#35832=DIRECTION('center_axis',(0.,1.,0.)) ;
#35833=DIRECTION('ref_axis',(0.,0.,1.)) ;
#35834=DIRECTION('',(1.,0.,0.)) ;
#35835=DIRECTION('center_axis',(0.,-1.,0.)) ;
#35836=DIRECTION('ref_axis',(0.,0.,-1.)) ;
#35837=DIRECTION('',(-1.,0.,0.)) ;
#35838=DIRECTION('center_axis',(0.,0.,1.)) ;
#35839=DIRECTION('ref_axis',(1.,0.,0.)) ;
#43759=CARTESIAN_POINT('',(0.,0.,0.)) ;
#43760=CARTESIAN_POINT('Origin',(-8.5,-22.,29.)) ;
#43761=CARTESIAN_POINT('',(-9.15,-22.,30.9)) ;
#43762=CARTESIAN_POINT('Origin',(-8.5,-22.,30.9)) ;
#43763=CARTESIAN_POINT('',(-9.15,-22.,31.)) ;
#43764=CARTESIAN_POINT('',(-9.15,-22.,29.)) ;
#43765=CARTESIAN_POINT('Origin',(-8.5,-22.,31.)) ;
#43766=CARTESIAN_POINT('Origin',(-8.5,-22.,29.)) ;
#43767=CARTESIAN_POINT('',(-9.15,-22.,27.)) ;
#43768=CARTESIAN_POINT('Origin',(-8.5,-22.,27.)) ;
#43769=CARTESIAN_POINT('',(-9.15,-22.,27.1)) ;
#43770=CARTESIAN_POINT('',(-9.15,-22.,29.)) ;
#43771=CARTESIAN_POINT('Origin',(-8.5,-22.,27.1)) ;
#43772=CARTESIAN_POINT('Origin',(-8.5,22.,29.)) ;
#43773=CARTESIAN_POINT('',(-9.15,22.,30.9)) ;
#43774=CARTESIAN_POINT('Origin',(-8.5,22.,30.9)) ;
#43775=CARTESIAN_POINT('',(-9.15,22.,31.)) ;
#43776=CARTESIAN_POINT('',(-9.15,22.,29.)) ;
#43777=CARTESIAN_POINT('Origin',(-8.5,22.,31.)) ;
#43778=CARTESIAN_POINT('Origin',(-8.5,22.,29.)) ;
#43779=CARTESIAN_POINT('',(-9.15,22.,27.)) ;
#43780=CARTESIAN_POINT('Origin',(-8.5,22.,27.)) ;
#43781=CARTESIAN_POINT('',(-9.15,22.,27.1)) ;
#43782=CARTESIAN_POINT('',(-9.15,22.,29.)) ;
#43783=CARTESIAN_POINT('Origin',(-8.5,22.,27.1)) ;
#43784=CARTESIAN_POINT('Origin',(8.5,-22.,29.)) ;
#43785=CARTESIAN_POINT('',(7.85,-22.,30.9)) ;
#43786=CARTESIAN_POINT('Origin',(8.5,-22.,30.9)) ;
#43787=CARTESIAN_POINT('',(7.85,-22.,31.)) ;
#43788=CARTESIAN_POINT('',(7.85,-22.,29.)) ;
#43789=CARTESIAN_POINT('Origin',(8.5,-22.,31.)) ;
#43790=CARTESIAN_POINT('Origin',(8.5,-22.,29.)) ;
#43791=CARTESIAN_POINT('',(7.85,-22.,27.)) ;
#43792=CARTESIAN_POINT('Origin',(8.5,-22.,27.)) ;
#43793=CARTESIAN_POINT('',(7.85,-22.,27.1)) ;
#43794=CARTESIAN_POINT('',(7.85,-22.,29.)) ;
#43795=CARTESIAN_POINT('Origin',(8.5,-22.,27.1)) ;
#43796=CARTESIAN_POINT('Origin',(-53.,0.,25.)) ;
#43797=CARTESIAN_POINT('',(-55.1424285285629,-20.4,27.1)) ;
#43798=CARTESIAN_POINT('',(-55.1424285285629,-23.6,27.1)) ;
#43799=CARTESIAN_POINT('',(-55.1424285285629,0.,27.1)) ;
#43800=CARTESIAN_POINT('',(-50.8575714714371,-23.6,27.1)) ;
#43801=CARTESIAN_POINT('Origin',(-53.,-23.6,25.)) ;
#43802=CARTESIAN_POINT('',(-50.8575714714371,-20.4,27.1)) ;
#43803=CARTESIAN_POINT('',(-50.8575714714371,0.,27.1)) ;
#43804=CARTESIAN_POINT('Origin',(-53.,-20.4,25.)) ;
#43805=CARTESIAN_POINT('Origin',(34.6,-22.,29.)) ;
#43806=CARTESIAN_POINT('',(34.6,-23.6,30.9)) ;
#43807=CARTESIAN_POINT('',(34.6,-23.6,27.1)) ;
#43808=CARTESIAN_POINT('',(34.6,-23.6,29.)) ;
#43809=CARTESIAN_POINT('',(34.6,-20.4,30.9)) ;
#43810=CARTESIAN_POINT('',(34.6,-22.,30.9)) ;
#43811=CARTESIAN_POINT('',(34.6,-20.4,27.1)) ;
#43812=CARTESIAN_POINT('',(34.6,-20.4,29.)) ;
#43813=CARTESIAN_POINT('',(34.6,-22.,27.1)) ;
#43814=CARTESIAN_POINT('Origin',(-10.5,-20.4,29.)) ;
#43815=CARTESIAN_POINT('',(-10.5,-20.4,27.1)) ;
#43816=CARTESIAN_POINT('',(-55.6,-20.4,30.9)) ;
#43817=CARTESIAN_POINT('',(-10.5,-20.4,30.9)) ;
#43818=CARTESIAN_POINT('',(-55.6,-20.4,27.1)) ;
#43819=CARTESIAN_POINT('',(-55.6,-20.4,29.)) ;
#43820=CARTESIAN_POINT('',(-10.5,-20.4,27.1)) ;
#43821=CARTESIAN_POINT('Origin',(-55.6,-22.,29.)) ;
#43822=CARTESIAN_POINT('',(-55.6,-23.6,30.9)) ;
#43823=CARTESIAN_POINT('',(-55.6,-22.,30.9)) ;
#43824=CARTESIAN_POINT('',(-55.6,-23.6,27.1)) ;
#43825=CARTESIAN_POINT('',(-55.6,-23.6,29.)) ;
#43826=CARTESIAN_POINT('',(-55.6,-22.,27.1)) ;
#43827=CARTESIAN_POINT('Origin',(-10.5,-22.,27.1)) ;
#43828=CARTESIAN_POINT('',(-10.5,-23.6,27.1)) ;
#43829=CARTESIAN_POINT('Origin',(-10.5,-22.,30.9)) ;
#43830=CARTESIAN_POINT('',(-10.5,-23.6,30.9)) ;
#43831=CARTESIAN_POINT('Origin',(-10.5,-22.,27.1)) ;
#43832=CARTESIAN_POINT('',(-10.5,-23.6,27.1)) ;
#43833=CARTESIAN_POINT('Origin',(-10.5,-23.6,29.)) ;
#43834=CARTESIAN_POINT('Origin',(8.5,22.,29.)) ;
#43835=CARTESIAN_POINT('',(7.85,22.,30.9)) ;
#43836=CARTESIAN_POINT('Origin',(8.5,22.,30.9)) ;
#43837=CARTESIAN_POINT('',(7.85,22.,31.)) ;
#43838=CARTESIAN_POINT('',(7.85,22.,29.)) ;
#43839=CARTESIAN_POINT('Origin',(8.5,22.,31.)) ;
#43840=CARTESIAN_POINT('Origin',(8.5,22.,29.)) ;
#43841=CARTESIAN_POINT('',(7.85,22.,27.)) ;
#43842=CARTESIAN_POINT('Origin',(8.5,22.,27.)) ;
#43843=CARTESIAN_POINT('',(7.85,22.,27.1)) ;
#43844=CARTESIAN_POINT('',(7.85,22.,29.)) ;
#43845=CARTESIAN_POINT('Origin',(8.5,22.,27.1)) ;
#43846=CARTESIAN_POINT('Origin',(-53.,0.,25.)) ;
#43847=CARTESIAN_POINT('',(-55.1424285285629,23.6,27.1)) ;
#43848=CARTESIAN_POINT('',(-55.1424285285629,20.4,27.1)) ;
#43849=CARTESIAN_POINT('',(-55.1424285285629,0.,27.1)) ;
#43850=CARTESIAN_POINT('',(-50.8575714714371,20.4,27.1)) ;
#43851=CARTESIAN_POINT('Origin',(-53.,20.4,25.)) ;
#43852=CARTESIAN_POINT('',(-50.8575714714371,23.6,27.1)) ;
#43853=CARTESIAN_POINT('',(-50.8575714714371,0.,27.1)) ;
#43854=CARTESIAN_POINT('Origin',(-53.,23.6,25.)) ;
#43855=CARTESIAN_POINT('Origin',(34.6,22.,29.)) ;
#43856=CARTESIAN_POINT('',(34.6,20.4,30.9)) ;
#43857=CARTESIAN_POINT('',(34.6,20.4,27.1)) ;
#43858=CARTESIAN_POINT('',(34.6,20.4,29.)) ;
#43859=CARTESIAN_POINT('',(34.6,23.6,30.9)) ;
#43860=CARTESIAN_POINT('',(34.6,22.,30.9)) ;
#43861=CARTESIAN_POINT('',(34.6,23.6,27.1)) ;
#43862=CARTESIAN_POINT('',(34.6,23.6,29.)) ;
#43863=CARTESIAN_POINT('',(34.6,22.,27.1)) ;
#43864=CARTESIAN_POINT('Origin',(-10.5,23.6,29.)) ;
#43865=CARTESIAN_POINT('',(-10.5,23.6,27.1)) ;
#43866=CARTESIAN_POINT('',(-55.6,23.6,30.9)) ;
#43867=CARTESIAN_POINT('',(-10.5,23.6,30.9)) ;
#43868=CARTESIAN_POINT('',(-55.6,23.6,27.1)) ;
#43869=CARTESIAN_POINT('',(-55.6,23.6,29.)) ;
#43870=CARTESIAN_POINT('',(-10.5,23.6,27.1)) ;
#43871=CARTESIAN_POINT('Origin',(-55.6,22.,29.)) ;
#43872=CARTESIAN_POINT('',(-55.6,20.4,30.9)) ;
#43873=CARTESIAN_POINT('',(-55.6,22.,30.9)) ;
#43874=CARTESIAN_POINT('',(-55.6,20.4,27.1)) ;
#43875=CARTESIAN_POINT('',(-55.6,20.4,29.)) ;
#43876=CARTESIAN_POINT('',(-55.6,22.,27.1)) ;
#43877=CARTESIAN_POINT('Origin',(-10.5,22.,27.1)) ;
#43878=CARTESIAN_POINT('',(-10.5,20.4,27.1)) ;
#43879=CARTESIAN_POINT('Origin',(-10.5,22.,30.9)) ;
#43880=CARTESIAN_POINT('',(-10.5,20.4,30.9)) ;
#43881=CARTESIAN_POINT('Origin',(-10.5,22.,27.1)) ;
#43882=CARTESIAN_POINT('',(-10.5,20.4,27.1)) ;
#43883=CARTESIAN_POINT('Origin',(-10.5,20.4,29.)) ;
#43884=CARTESIAN_POINT('Origin',(-53.,0.,90.)) ;
#43885=CARTESIAN_POINT('',(-54.28,-4.8,90.)) ;
#43886=CARTESIAN_POINT('Origin',(-53.,-4.8,90.)) ;
#43887=CARTESIAN_POINT('',(-54.28,-4.,90.)) ;
#43888=CARTESIAN_POINT('',(-54.28,0.,90.)) ;
#43889=CARTESIAN_POINT('Origin',(-53.,-4.,90.)) ;
#43890=CARTESIAN_POINT('Origin',(-53.,0.,90.)) ;
#43891=CARTESIAN_POINT('',(-54.28,4.,90.)) ;
#43892=CARTESIAN_POINT('Origin',(-53.,4.,90.)) ;
#43893=CARTESIAN_POINT('',(-54.28,4.8,90.)) ;
#43894=CARTESIAN_POINT('',(-54.28,0.,90.)) ;
#43895=CARTESIAN_POINT('Origin',(-53.,4.8,90.)) ;
#43896=CARTESIAN_POINT('Origin',(-21.92,-21.92,49.5)) ;
#43897=CARTESIAN_POINT('',(-23.12,-21.92,31.)) ;
#43898=CARTESIAN_POINT('Origin',(-21.92,-21.92,31.)) ;
#43899=CARTESIAN_POINT('',(-23.12,-21.92,68.)) ;
#43900=CARTESIAN_POINT('',(-23.12,-21.92,49.5)) ;
#43901=CARTESIAN_POINT('Origin',(-21.92,-21.92,68.)) ;
#43902=CARTESIAN_POINT('Origin',(-21.92,-21.92,49.5)) ;
#43903=CARTESIAN_POINT('',(-23.42,-21.92,68.)) ;
#43904=CARTESIAN_POINT('Origin',(-21.92,-21.92,68.)) ;
#43905=CARTESIAN_POINT('',(-23.42,-21.92,31.)) ;
#43906=CARTESIAN_POINT('',(-23.42,-21.92,49.5)) ;
#43907=CARTESIAN_POINT('Origin',(-21.92,-21.92,31.)) ;
#43908=CARTESIAN_POINT('Origin',(-21.92,-21.92,68.)) ;
#43909=CARTESIAN_POINT('Origin',(-10.5,-22.,31.)) ;
#43910=CARTESIAN_POINT('',(35.,-24.,31.)) ;
#43911=CARTESIAN_POINT('',(35.,-20.,31.)) ;
#43912=CARTESIAN_POINT('',(35.,-22.,31.)) ;
#43913=CARTESIAN_POINT('',(-56.,-20.,31.)) ;
#43914=CARTESIAN_POINT('',(-10.5,-20.,31.)) ;
#43915=CARTESIAN_POINT('',(-56.,-24.,31.)) ;
#43916=CARTESIAN_POINT('',(-56.,-22.,31.)) ;
#43917=CARTESIAN_POINT('',(-50.,-24.,31.)) ;
#43918=CARTESIAN_POINT('',(-31.75,-24.,31.)) ;
#43919=CARTESIAN_POINT('',(-10.5,-24.,31.)) ;
#43920=CARTESIAN_POINT('',(20.42,-21.92,31.)) ;
#43921=CARTESIAN_POINT('Origin',(21.92,-21.92,31.)) ;
#43922=CARTESIAN_POINT('Origin',(21.92,-21.92,49.5)) ;
#43923=CARTESIAN_POINT('',(20.72,-21.92,31.)) ;
#43924=CARTESIAN_POINT('Origin',(21.92,-21.92,31.)) ;
#43925=CARTESIAN_POINT('',(20.72,-21.92,68.)) ;
#43926=CARTESIAN_POINT('',(20.72,-21.92,49.5)) ;
#43927=CARTESIAN_POINT('Origin',(21.92,-21.92,68.)) ;
#43928=CARTESIAN_POINT('Origin',(21.92,-21.92,49.5)) ;
#43929=CARTESIAN_POINT('',(20.42,-21.92,68.)) ;
#43930=CARTESIAN_POINT('Origin',(21.92,-21.92,68.)) ;
#43931=CARTESIAN_POINT('',(20.42,-21.92,49.5)) ;
#43932=CARTESIAN_POINT('Origin',(21.92,-21.92,68.)) ;
#43933=CARTESIAN_POINT('Origin',(-10.5,-22.,31.)) ;
#43934=CARTESIAN_POINT('Origin',(22.,-20.4,13.8)) ;
#43935=CARTESIAN_POINT('',(20.4,-20.4,27.)) ;
#43936=CARTESIAN_POINT('',(23.6,-20.4,27.)) ;
#43937=CARTESIAN_POINT('',(5.75,-20.4,27.)) ;
#43938=CARTESIAN_POINT('',(20.4,-20.4,0.6)) ;
#43939=CARTESIAN_POINT('',(20.4,-20.4,13.8)) ;
#43940=CARTESIAN_POINT('',(23.6,-20.4,0.6)) ;
#43941=CARTESIAN_POINT('',(22.,-20.4,0.6)) ;
#43942=CARTESIAN_POINT('',(23.6,-20.4,13.8)) ;
#43943=CARTESIAN_POINT('Origin',(23.6,-22.,13.8)) ;
#43944=CARTESIAN_POINT('',(23.6,-23.6,27.)) ;
#43945=CARTESIAN_POINT('',(23.6,-22.,27.)) ;
#43946=CARTESIAN_POINT('',(23.6,-23.6,0.6)) ;
#43947=CARTESIAN_POINT('',(23.6,-22.,0.6)) ;
#43948=CARTESIAN_POINT('',(23.6,-23.6,13.8)) ;
#43949=CARTESIAN_POINT('Origin',(22.,-23.6,13.8)) ;
#43950=CARTESIAN_POINT('',(20.4,-23.6,27.)) ;
#43951=CARTESIAN_POINT('',(5.75,-23.6,27.)) ;
#43952=CARTESIAN_POINT('',(20.4,-23.6,0.6)) ;
#43953=CARTESIAN_POINT('',(22.,-23.6,0.6)) ;
#43954=CARTESIAN_POINT('',(20.4,-23.6,13.8)) ;
#43955=CARTESIAN_POINT('Origin',(20.4,-22.,13.8)) ;
#43956=CARTESIAN_POINT('',(20.4,-22.,27.)) ;
#43957=CARTESIAN_POINT('',(20.4,-22.,0.6)) ;
#43958=CARTESIAN_POINT('Origin',(22.,-22.,0.6)) ;
#43959=CARTESIAN_POINT('',(24.,-20.,0.6)) ;
#43960=CARTESIAN_POINT('',(24.,-24.,0.6)) ;
#43961=CARTESIAN_POINT('',(24.,-22.,0.6)) ;
#43962=CARTESIAN_POINT('',(20.,-24.,0.6)) ;
#43963=CARTESIAN_POINT('',(22.,-24.,0.6)) ;
#43964=CARTESIAN_POINT('',(20.,-20.,0.6)) ;
#43965=CARTESIAN_POINT('',(20.,-22.,0.6)) ;
#43966=CARTESIAN_POINT('',(22.,-20.,0.6)) ;
#43967=CARTESIAN_POINT('Origin',(20.,-22.,13.8)) ;
#43968=CARTESIAN_POINT('',(20.,-20.,27.)) ;
#43969=CARTESIAN_POINT('',(20.,-20.,13.8)) ;
#43970=CARTESIAN_POINT('',(20.,-24.,27.)) ;
#43971=CARTESIAN_POINT('',(20.,-24.,13.8)) ;
#43972=CARTESIAN_POINT('',(20.,-22.,27.)) ;
#43973=CARTESIAN_POINT('Origin',(24.,-22.,13.8)) ;
#43974=CARTESIAN_POINT('',(24.,-24.,27.)) ;
#43975=CARTESIAN_POINT('',(24.,-24.,13.8)) ;
#43976=CARTESIAN_POINT('',(24.,-20.,27.)) ;
#43977=CARTESIAN_POINT('',(24.,-20.,13.8)) ;
#43978=CARTESIAN_POINT('',(24.,-22.,27.)) ;
#43979=CARTESIAN_POINT('Origin',(-10.5,-22.,27.)) ;
#43980=CARTESIAN_POINT('',(-50.,-24.,27.)) ;
#43981=CARTESIAN_POINT('',(-10.5,-24.,27.)) ;
#43982=CARTESIAN_POINT('',(-50.7639320225002,-24.,27.)) ;
#43983=CARTESIAN_POINT('',(-31.75,-24.,27.)) ;
#43984=CARTESIAN_POINT('',(-50.7639320225002,-20.,27.)) ;
#43985=CARTESIAN_POINT('',(-50.7639320225002,0.,27.)) ;
#43986=CARTESIAN_POINT('',(-10.5,-20.,27.)) ;
#43987=CARTESIAN_POINT('Origin',(-10.5,-22.,27.)) ;
#43988=CARTESIAN_POINT('Origin',(-10.5,22.,27.)) ;
#43989=CARTESIAN_POINT('',(-55.2360679774998,20.,27.)) ;
#43990=CARTESIAN_POINT('',(-55.2360679774998,24.,27.)) ;
#43991=CARTESIAN_POINT('',(-55.2360679774998,0.,27.)) ;
#43992=CARTESIAN_POINT('',(-56.,20.,27.)) ;
#43993=CARTESIAN_POINT('',(-10.5,20.,27.)) ;
#43994=CARTESIAN_POINT('',(-56.,24.,27.)) ;
#43995=CARTESIAN_POINT('',(-56.,22.,27.)) ;
#43996=CARTESIAN_POINT('',(-31.75,24.,27.)) ;
#43997=CARTESIAN_POINT('Origin',(-10.5,22.,31.)) ;
#43998=CARTESIAN_POINT('',(20.72,21.92,31.)) ;
#43999=CARTESIAN_POINT('Origin',(21.92,21.92,31.)) ;
#44000=CARTESIAN_POINT('Origin',(-10.5,22.,27.)) ;
#44001=CARTESIAN_POINT('',(24.,20.,27.)) ;
#44002=CARTESIAN_POINT('',(24.,24.,27.)) ;
#44003=CARTESIAN_POINT('',(24.,22.,27.)) ;
#44004=CARTESIAN_POINT('',(35.,24.,27.)) ;
#44005=CARTESIAN_POINT('',(-10.5,24.,27.)) ;
#44006=CARTESIAN_POINT('',(35.,20.,27.)) ;
#44007=CARTESIAN_POINT('',(35.,22.,27.)) ;
#44008=CARTESIAN_POINT('',(-10.5,20.,27.)) ;
#44009=CARTESIAN_POINT('Origin',(-10.5,20.,29.)) ;
#44010=CARTESIAN_POINT('',(-50.7639320225002,20.,27.)) ;
#44011=CARTESIAN_POINT('Origin',(-53.,20.,25.)) ;
#44012=CARTESIAN_POINT('',(20.,20.,27.)) ;
#44013=CARTESIAN_POINT('',(-10.5,20.,27.)) ;
#44014=CARTESIAN_POINT('',(20.,20.,0.6)) ;
#44015=CARTESIAN_POINT('',(20.,20.,13.8)) ;
#44016=CARTESIAN_POINT('',(24.,20.,0.6)) ;
#44017=CARTESIAN_POINT('',(22.,20.,0.6)) ;
#44018=CARTESIAN_POINT('',(24.,20.,13.8)) ;
#44019=CARTESIAN_POINT('',(35.,20.,31.)) ;
#44020=CARTESIAN_POINT('',(35.,20.,29.)) ;
#44021=CARTESIAN_POINT('',(-56.,20.,31.)) ;
#44022=CARTESIAN_POINT('',(-10.5,20.,31.)) ;
#44023=CARTESIAN_POINT('',(-56.,20.,29.)) ;
#44024=CARTESIAN_POINT('Origin',(-10.5,24.,29.)) ;
#44025=CARTESIAN_POINT('',(-50.,24.,31.)) ;
#44026=CARTESIAN_POINT('',(-50.,24.,27.)) ;
#44027=CARTESIAN_POINT('',(-50.,24.,43.3)) ;
#44028=CARTESIAN_POINT('',(35.,24.,31.)) ;
#44029=CARTESIAN_POINT('',(-10.5,24.,31.)) ;
#44030=CARTESIAN_POINT('',(35.,24.,29.)) ;
#44031=CARTESIAN_POINT('',(24.,24.,0.6)) ;
#44032=CARTESIAN_POINT('',(24.,24.,13.8)) ;
#44033=CARTESIAN_POINT('',(20.,24.,0.6)) ;
#44034=CARTESIAN_POINT('',(22.,24.,0.6)) ;
#44035=CARTESIAN_POINT('',(20.,24.,27.)) ;
#44036=CARTESIAN_POINT('',(20.,24.,13.8)) ;
#44037=CARTESIAN_POINT('',(-10.5,24.,27.)) ;
#44038=CARTESIAN_POINT('Origin',(35.,22.,29.)) ;
#44039=CARTESIAN_POINT('',(35.,22.,31.)) ;
#44040=CARTESIAN_POINT('Origin',(-53.,24.,43.3)) ;
#44041=CARTESIAN_POINT('',(-50.7639320225002,24.,27.)) ;
#44042=CARTESIAN_POINT('',(-31.75,24.,27.)) ;
#44043=CARTESIAN_POINT('',(-50.1715728752538,24.,26.)) ;
#44044=CARTESIAN_POINT('Origin',(-53.,24.,25.)) ;
#44045=CARTESIAN_POINT('',(-50.,24.,26.)) ;
#44046=CARTESIAN_POINT('',(-53.,24.,26.)) ;
#44047=CARTESIAN_POINT('',(-50.,24.,43.3)) ;
#44048=CARTESIAN_POINT('Origin',(-53.,24.,43.3)) ;
#44049=CARTESIAN_POINT('',(-56.,24.,26.)) ;
#44050=CARTESIAN_POINT('',(-56.,24.,43.3)) ;
#44051=CARTESIAN_POINT('',(-55.8284271247462,24.,26.)) ;
#44052=CARTESIAN_POINT('',(-53.,24.,26.)) ;
#44053=CARTESIAN_POINT('Origin',(-53.,24.,25.)) ;
#44054=CARTESIAN_POINT('Origin',(-53.,0.,26.)) ;
#44055=CARTESIAN_POINT('',(-50.1715728752538,-24.,26.)) ;
#44056=CARTESIAN_POINT('',(-50.1715728752538,0.,26.)) ;
#44057=CARTESIAN_POINT('',(-50.,-24.,26.)) ;
#44058=CARTESIAN_POINT('',(-53.,-24.,26.)) ;
#44059=CARTESIAN_POINT('',(-50.,0.,26.)) ;
#44060=CARTESIAN_POINT('Origin',(-53.,0.,22.)) ;
#44061=CARTESIAN_POINT('',(-50.4,-24.4,22.)) ;
#44062=CARTESIAN_POINT('',(-55.6,-24.4,22.)) ;
#44063=CARTESIAN_POINT('',(-53.,-24.4,22.)) ;
#44064=CARTESIAN_POINT('',(-50.4,-29.6,22.)) ;
#44065=CARTESIAN_POINT('',(-50.4,-13.5,22.)) ;
#44066=CARTESIAN_POINT('',(-55.6,-29.6,22.)) ;
#44067=CARTESIAN_POINT('',(-53.,-29.6,22.)) ;
#44068=CARTESIAN_POINT('',(-55.6,-13.5,22.)) ;
#44069=CARTESIAN_POINT('Origin',(-53.,0.,22.)) ;
#44070=CARTESIAN_POINT('',(-50.4,29.6,22.)) ;
#44071=CARTESIAN_POINT('',(-55.6,29.6,22.)) ;
#44072=CARTESIAN_POINT('',(-53.,29.6,22.)) ;
#44073=CARTESIAN_POINT('',(-50.4,24.4,22.)) ;
#44074=CARTESIAN_POINT('',(-50.4,13.5,22.)) ;
#44075=CARTESIAN_POINT('',(-55.6,24.4,22.)) ;
#44076=CARTESIAN_POINT('',(-53.,24.4,22.)) ;
#44077=CARTESIAN_POINT('',(-55.6,13.5,22.)) ;
#44078=CARTESIAN_POINT('Origin',(-53.,0.,22.)) ;
#44079=CARTESIAN_POINT('',(-50.,24.,22.)) ;
#44080=CARTESIAN_POINT('',(-56.,24.,22.)) ;
#44081=CARTESIAN_POINT('',(-53.,24.,22.)) ;
#44082=CARTESIAN_POINT('',(-50.,-24.,22.)) ;
#44083=CARTESIAN_POINT('',(-50.,0.,22.)) ;
#44084=CARTESIAN_POINT('',(-56.,-24.,22.)) ;
#44085=CARTESIAN_POINT('',(-53.,-24.,22.)) ;
#44086=CARTESIAN_POINT('',(-56.,0.,22.)) ;
#44087=CARTESIAN_POINT('Origin',(-53.,0.,26.)) ;
#44088=CARTESIAN_POINT('',(-56.,-24.,26.)) ;
#44089=CARTESIAN_POINT('',(-56.,0.,26.)) ;
#44090=CARTESIAN_POINT('',(-55.8284271247462,-24.,26.)) ;
#44091=CARTESIAN_POINT('',(-53.,-24.,26.)) ;
#44092=CARTESIAN_POINT('',(-55.8284271247462,0.,26.)) ;
#44093=CARTESIAN_POINT('Origin',(-53.,30.,43.3)) ;
#44094=CARTESIAN_POINT('',(-56.,30.,86.)) ;
#44095=CARTESIAN_POINT('',(-56.,30.,25.)) ;
#44096=CARTESIAN_POINT('',(-56.,30.,43.3)) ;
#44097=CARTESIAN_POINT('',(-50.,30.,86.)) ;
#44098=CARTESIAN_POINT('',(-53.,30.,86.)) ;
#44099=CARTESIAN_POINT('',(-50.,30.,25.)) ;
#44100=CARTESIAN_POINT('',(-50.,30.,43.3)) ;
#44101=CARTESIAN_POINT('Origin',(-53.,30.,25.)) ;
#44102=CARTESIAN_POINT('Origin',(-53.,30.,43.3)) ;
#44103=CARTESIAN_POINT('',(-50.,30.,0.600000000000001)) ;
#44104=CARTESIAN_POINT('',(-50.,30.,43.3)) ;
#44105=CARTESIAN_POINT('',(-56.,30.,0.600000000000001)) ;
#44106=CARTESIAN_POINT('',(-53.,30.,0.600000000000001)) ;
#44107=CARTESIAN_POINT('',(-56.,30.,43.3)) ;
#44108=CARTESIAN_POINT('Origin',(-53.,30.,25.)) ;
#44109=CARTESIAN_POINT('Origin',(-56.,27.,43.3)) ;
#44110=CARTESIAN_POINT('',(-56.,-4.,82.)) ;
#44111=CARTESIAN_POINT('',(-56.,-4.,86.)) ;
#44112=CARTESIAN_POINT('',(-56.,-4.,65.65)) ;
#44113=CARTESIAN_POINT('',(-56.,4.,86.)) ;
#44114=CARTESIAN_POINT('',(-56.,27.,86.)) ;
#44115=CARTESIAN_POINT('',(-56.,4.,82.)) ;
#44116=CARTESIAN_POINT('',(-56.,4.,65.65)) ;
#44117=CARTESIAN_POINT('',(-56.,4.8,82.)) ;
#44118=CARTESIAN_POINT('',(-56.,15.7,82.)) ;
#44119=CARTESIAN_POINT('',(-56.,4.8,86.)) ;
#44120=CARTESIAN_POINT('',(-56.,4.8,65.65)) ;
#44121=CARTESIAN_POINT('',(-56.,27.,86.)) ;
#44122=CARTESIAN_POINT('',(-56.,24.,0.600000000000001)) ;
#44123=CARTESIAN_POINT('',(-56.,27.,0.600000000000001)) ;
#44124=CARTESIAN_POINT('',(-56.,24.,43.3)) ;
#44125=CARTESIAN_POINT('',(-56.,-24.,0.600000000000001)) ;
#44126=CARTESIAN_POINT('',(-56.,-24.,43.3)) ;
#44127=CARTESIAN_POINT('',(-56.,-30.,0.600000000000001)) ;
#44128=CARTESIAN_POINT('',(-56.,-27.,0.600000000000001)) ;
#44129=CARTESIAN_POINT('',(-56.,-30.,25.)) ;
#44130=CARTESIAN_POINT('',(-56.,-30.,43.3)) ;
#44131=CARTESIAN_POINT('',(-56.,-30.,86.)) ;
#44132=CARTESIAN_POINT('',(-56.,-30.,43.3)) ;
#44133=CARTESIAN_POINT('',(-56.,-4.8,86.)) ;
#44134=CARTESIAN_POINT('',(-56.,27.,86.)) ;
#44135=CARTESIAN_POINT('',(-56.,-4.8,82.)) ;
#44136=CARTESIAN_POINT('',(-56.,-4.8,65.65)) ;
#44137=CARTESIAN_POINT('',(-56.,11.3,82.)) ;
#44138=CARTESIAN_POINT('',(-56.,24.,80.)) ;
#44139=CARTESIAN_POINT('',(-56.,24.,31.)) ;
#44140=CARTESIAN_POINT('',(-56.,24.,43.3)) ;
#44141=CARTESIAN_POINT('',(-56.,-24.,80.)) ;
#44142=CARTESIAN_POINT('',(-56.,0.,80.)) ;
#44143=CARTESIAN_POINT('',(-56.,-24.,43.3)) ;
#44144=CARTESIAN_POINT('',(-56.,-20.,27.)) ;
#44145=CARTESIAN_POINT('',(-56.,-20.,29.)) ;
#44146=CARTESIAN_POINT('',(-56.,-24.,27.)) ;
#44147=CARTESIAN_POINT('',(-56.,-22.,27.)) ;
#44148=CARTESIAN_POINT('',(-56.,-24.,43.3)) ;
#44149=CARTESIAN_POINT('',(-56.,22.,31.)) ;
#44150=CARTESIAN_POINT('Origin',(-53.,-30.,43.3)) ;
#44151=CARTESIAN_POINT('',(-50.,-30.,25.)) ;
#44152=CARTESIAN_POINT('Origin',(-53.,-30.,25.)) ;
#44153=CARTESIAN_POINT('',(-50.,-30.,86.)) ;
#44154=CARTESIAN_POINT('',(-50.,-30.,43.3)) ;
#44155=CARTESIAN_POINT('',(-53.,-30.,86.)) ;
#44156=CARTESIAN_POINT('Origin',(-53.,24.,43.3)) ;
#44157=CARTESIAN_POINT('',(-50.,24.,0.600000000000001)) ;
#44158=CARTESIAN_POINT('',(-53.,24.,0.600000000000001)) ;
#44159=CARTESIAN_POINT('',(-50.,24.,43.3)) ;
#44160=CARTESIAN_POINT('Origin',(-53.,-24.,43.3)) ;
#44161=CARTESIAN_POINT('',(-50.,-24.,0.600000000000001)) ;
#44162=CARTESIAN_POINT('',(-50.,-24.,43.3)) ;
#44163=CARTESIAN_POINT('',(-53.,-24.,0.600000000000001)) ;
#44164=CARTESIAN_POINT('Origin',(-55.6,27.,43.3)) ;
#44165=CARTESIAN_POINT('',(-55.6,24.4,0.600000000000001)) ;
#44166=CARTESIAN_POINT('',(-55.6,24.4,43.3)) ;
#44167=CARTESIAN_POINT('',(-55.6,29.6,0.600000000000001)) ;
#44168=CARTESIAN_POINT('',(-55.6,27.,0.600000000000001)) ;
#44169=CARTESIAN_POINT('',(-55.6,29.6,43.3)) ;
#44170=CARTESIAN_POINT('Origin',(-53.,29.6,43.3)) ;
#44171=CARTESIAN_POINT('',(-50.4,29.6,0.600000000000001)) ;
#44172=CARTESIAN_POINT('',(-53.,29.6,0.600000000000001)) ;
#44173=CARTESIAN_POINT('',(-50.4,29.6,43.3)) ;
#44174=CARTESIAN_POINT('Origin',(-55.6,-27.,43.3)) ;
#44175=CARTESIAN_POINT('',(-55.6,-29.6,0.600000000000001)) ;
#44176=CARTESIAN_POINT('',(-55.6,-29.6,43.3)) ;
#44177=CARTESIAN_POINT('',(-55.6,-24.4,0.600000000000001)) ;
#44178=CARTESIAN_POINT('',(-55.6,-27.,0.600000000000001)) ;
#44179=CARTESIAN_POINT('',(-55.6,-24.4,43.3)) ;
#44180=CARTESIAN_POINT('Origin',(-53.,-24.4,43.3)) ;
#44181=CARTESIAN_POINT('',(-50.4,-24.4,0.600000000000001)) ;
#44182=CARTESIAN_POINT('',(-53.,-24.4,0.600000000000001)) ;
#44183=CARTESIAN_POINT('',(-50.4,-24.4,43.3)) ;
#44184=CARTESIAN_POINT('Origin',(-53.,27.,0.600000000000001)) ;
#44185=CARTESIAN_POINT('',(-50.,27.,0.600000000000001)) ;
#44186=CARTESIAN_POINT('',(-50.4,24.4,0.600000000000001)) ;
#44187=CARTESIAN_POINT('',(-53.,24.4,0.600000000000001)) ;
#44188=CARTESIAN_POINT('',(-50.4,27.,0.600000000000001)) ;
#44189=CARTESIAN_POINT('Origin',(-53.,27.,86.)) ;
#44190=CARTESIAN_POINT('',(-50.,4.8,86.)) ;
#44191=CARTESIAN_POINT('',(-53.,4.8,86.)) ;
#44192=CARTESIAN_POINT('',(-50.,27.,86.)) ;
#44193=CARTESIAN_POINT('Origin',(-53.,30.,43.3)) ;
#44194=CARTESIAN_POINT('',(-55.6,30.,25.)) ;
#44195=CARTESIAN_POINT('Origin',(-53.,30.,25.)) ;
#44196=CARTESIAN_POINT('Origin',(-53.,-30.,43.3)) ;
#44197=CARTESIAN_POINT('',(-55.6,-30.,25.)) ;
#44198=CARTESIAN_POINT('Origin',(-53.,-30.,25.)) ;
#44199=CARTESIAN_POINT('Origin',(-53.,-27.,0.600000000000001)) ;
#44200=CARTESIAN_POINT('',(-50.,-30.,0.600000000000001)) ;
#44201=CARTESIAN_POINT('',(-50.,-27.,0.600000000000001)) ;
#44202=CARTESIAN_POINT('',(-53.,-30.,0.600000000000001)) ;
#44203=CARTESIAN_POINT('',(-50.4,-29.6,0.600000000000001)) ;
#44204=CARTESIAN_POINT('',(-53.,-29.6,0.600000000000001)) ;
#44205=CARTESIAN_POINT('',(-50.4,-27.,0.600000000000001)) ;
#44206=CARTESIAN_POINT('Origin',(-53.,0.,80.)) ;
#44207=CARTESIAN_POINT('',(-50.,24.,80.)) ;
#44208=CARTESIAN_POINT('',(-53.,24.,80.)) ;
#44209=CARTESIAN_POINT('',(-50.,-24.,80.)) ;
#44210=CARTESIAN_POINT('',(-50.,0.,80.)) ;
#44211=CARTESIAN_POINT('',(-53.,-24.,80.)) ;
#44212=CARTESIAN_POINT('Origin',(-53.,24.,43.3)) ;
#44213=CARTESIAN_POINT('',(-31.75,24.,31.)) ;
#44214=CARTESIAN_POINT('',(-50.,24.,43.3)) ;
#44215=CARTESIAN_POINT('Origin',(-53.,-30.,43.3)) ;
#44216=CARTESIAN_POINT('',(-50.,-30.,43.3)) ;
#44217=CARTESIAN_POINT('Origin',(-53.,-30.,25.)) ;
#44218=CARTESIAN_POINT('Origin',(-53.,24.4,43.3)) ;
#44219=CARTESIAN_POINT('',(-50.4,24.4,43.3)) ;
#44220=CARTESIAN_POINT('Origin',(-50.4,27.,43.3)) ;
#44221=CARTESIAN_POINT('Origin',(-53.,-29.6,43.3)) ;
#44222=CARTESIAN_POINT('',(-50.4,-29.6,43.3)) ;
#44223=CARTESIAN_POINT('Origin',(-50.4,-27.,43.3)) ;
#44224=CARTESIAN_POINT('Origin',(-53.,43.,25.)) ;
#44225=CARTESIAN_POINT('',(-56.,43.,25.)) ;
#44226=CARTESIAN_POINT('Origin',(-53.,43.,25.)) ;
#44227=CARTESIAN_POINT('',(-55.6,43.,25.)) ;
#44228=CARTESIAN_POINT('Origin',(-53.,43.,25.)) ;
#44229=CARTESIAN_POINT('Origin',(-53.,-43.,25.)) ;
#44230=CARTESIAN_POINT('',(-56.,-43.,25.)) ;
#44231=CARTESIAN_POINT('Origin',(-53.,-43.,25.)) ;
#44232=CARTESIAN_POINT('',(-55.6,-43.,25.)) ;
#44233=CARTESIAN_POINT('Origin',(-53.,-43.,25.)) ;
#44234=CARTESIAN_POINT('Origin',(-53.,0.,25.)) ;
#44235=CARTESIAN_POINT('',(-56.,0.,25.)) ;
#44236=CARTESIAN_POINT('Origin',(-53.,0.,25.)) ;
#44237=CARTESIAN_POINT('',(-56.,0.,25.)) ;
#44238=CARTESIAN_POINT('Origin',(-53.,0.,25.)) ;
#44239=CARTESIAN_POINT('',(-55.6,0.,25.)) ;
#44240=CARTESIAN_POINT('Origin',(-53.,0.,25.)) ;
#44241=CARTESIAN_POINT('',(-55.6,0.,25.)) ;
#44242=CARTESIAN_POINT('Origin',(-53.,27.,86.)) ;
#44243=CARTESIAN_POINT('',(-50.,-4.,86.)) ;
#44244=CARTESIAN_POINT('',(-53.,-4.,86.)) ;
#44245=CARTESIAN_POINT('',(-50.,4.,86.)) ;
#44246=CARTESIAN_POINT('',(-50.,27.,86.)) ;
#44247=CARTESIAN_POINT('',(-53.,4.,86.)) ;
#44248=CARTESIAN_POINT('Origin',(-49.,4.4,88.)) ;
#44249=CARTESIAN_POINT('',(-49.,4.,94.)) ;
#44250=CARTESIAN_POINT('',(-49.,4.,82.)) ;
#44251=CARTESIAN_POINT('',(-49.,4.,88.)) ;
#44252=CARTESIAN_POINT('',(-49.,4.8,82.)) ;
#44253=CARTESIAN_POINT('',(-49.,4.4,82.)) ;
#44254=CARTESIAN_POINT('',(-49.,4.8,94.)) ;
#44255=CARTESIAN_POINT('',(-49.,4.8,88.)) ;
#44256=CARTESIAN_POINT('',(-49.,4.4,94.)) ;
#44257=CARTESIAN_POINT('Origin',(-57.,4.4,88.)) ;
#44258=CARTESIAN_POINT('',(-57.,4.8,94.)) ;
#44259=CARTESIAN_POINT('',(-57.,4.8,82.)) ;
#44260=CARTESIAN_POINT('',(-57.,4.8,88.)) ;
#44261=CARTESIAN_POINT('',(-57.,4.,82.)) ;
#44262=CARTESIAN_POINT('',(-57.,4.4,82.)) ;
#44263=CARTESIAN_POINT('',(-57.,4.,94.)) ;
#44264=CARTESIAN_POINT('',(-57.,4.,88.)) ;
#44265=CARTESIAN_POINT('',(-57.,4.4,94.)) ;
#44266=CARTESIAN_POINT('Origin',(-53.,4.4,94.)) ;
#44267=CARTESIAN_POINT('',(-53.,4.8,94.)) ;
#44268=CARTESIAN_POINT('',(-53.,4.,94.)) ;
#44269=CARTESIAN_POINT('Origin',(-53.,4.4,82.)) ;
#44270=CARTESIAN_POINT('',(-50.,4.8,82.)) ;
#44271=CARTESIAN_POINT('',(-50.,4.,82.)) ;
#44272=CARTESIAN_POINT('',(-50.,15.7,82.)) ;
#44273=CARTESIAN_POINT('',(-53.,4.8,82.)) ;
#44274=CARTESIAN_POINT('',(-53.,4.,82.)) ;
#44275=CARTESIAN_POINT('Origin',(-53.,4.4,82.)) ;
#44276=CARTESIAN_POINT('',(-53.,4.,82.)) ;
#44277=CARTESIAN_POINT('',(-53.,4.8,82.)) ;
#44278=CARTESIAN_POINT('Origin',(-53.,4.,88.)) ;
#44279=CARTESIAN_POINT('',(-50.,4.,65.65)) ;
#44280=CARTESIAN_POINT('Origin',(-53.,4.8,88.)) ;
#44281=CARTESIAN_POINT('',(-50.,4.8,65.65)) ;
#44282=CARTESIAN_POINT('Origin',(-10.5,22.,27.)) ;
#44283=CARTESIAN_POINT('',(20.4,23.6,27.)) ;
#44284=CARTESIAN_POINT('',(23.6,23.6,27.)) ;
#44285=CARTESIAN_POINT('',(5.75,23.6,27.)) ;
#44286=CARTESIAN_POINT('',(23.6,20.4,27.)) ;
#44287=CARTESIAN_POINT('',(23.6,22.,27.)) ;
#44288=CARTESIAN_POINT('',(20.4,20.4,27.)) ;
#44289=CARTESIAN_POINT('',(5.75,20.4,27.)) ;
#44290=CARTESIAN_POINT('',(20.4,22.,27.)) ;
#44291=CARTESIAN_POINT('Origin',(-10.5,22.,27.)) ;
#44292=CARTESIAN_POINT('',(20.,22.,27.)) ;
#44293=CARTESIAN_POINT('',(-50.7639320225002,0.,27.)) ;
#44294=CARTESIAN_POINT('Origin',(24.,22.,13.8)) ;
#44295=CARTESIAN_POINT('',(24.,22.,0.6)) ;
#44296=CARTESIAN_POINT('Origin',(20.,22.,13.8)) ;
#44297=CARTESIAN_POINT('',(20.,22.,0.6)) ;
#44298=CARTESIAN_POINT('Origin',(22.,22.,0.6)) ;
#44299=CARTESIAN_POINT('',(20.4,20.4,0.6)) ;
#44300=CARTESIAN_POINT('',(23.6,20.4,0.6)) ;
#44301=CARTESIAN_POINT('',(22.,20.4,0.6)) ;
#44302=CARTESIAN_POINT('',(23.6,23.6,0.6)) ;
#44303=CARTESIAN_POINT('',(23.6,22.,0.6)) ;
#44304=CARTESIAN_POINT('',(20.4,23.6,0.6)) ;
#44305=CARTESIAN_POINT('',(22.,23.6,0.6)) ;
#44306=CARTESIAN_POINT('',(20.4,22.,0.6)) ;
#44307=CARTESIAN_POINT('Origin',(20.4,22.,13.8)) ;
#44308=CARTESIAN_POINT('',(20.4,20.4,13.8)) ;
#44309=CARTESIAN_POINT('',(20.4,23.6,13.8)) ;
#44310=CARTESIAN_POINT('Origin',(22.,20.4,13.8)) ;
#44311=CARTESIAN_POINT('',(23.6,20.4,13.8)) ;
#44312=CARTESIAN_POINT('Origin',(23.6,22.,13.8)) ;
#44313=CARTESIAN_POINT('',(23.6,23.6,13.8)) ;
#44314=CARTESIAN_POINT('Origin',(22.,23.6,13.8)) ;
#44315=CARTESIAN_POINT('Origin',(-10.5,22.,31.)) ;
#44316=CARTESIAN_POINT('',(-23.12,21.92,31.)) ;
#44317=CARTESIAN_POINT('Origin',(-21.92,21.92,31.)) ;
#44318=CARTESIAN_POINT('Origin',(21.92,21.92,68.)) ;
#44319=CARTESIAN_POINT('',(20.42,21.92,68.)) ;
#44320=CARTESIAN_POINT('Origin',(21.92,21.92,68.)) ;
#44321=CARTESIAN_POINT('',(20.72,21.92,68.)) ;
#44322=CARTESIAN_POINT('Origin',(21.92,21.92,68.)) ;
#44323=CARTESIAN_POINT('Origin',(21.92,21.92,49.5)) ;
#44324=CARTESIAN_POINT('',(20.42,21.92,31.)) ;
#44325=CARTESIAN_POINT('',(20.42,21.92,49.5)) ;
#44326=CARTESIAN_POINT('Origin',(21.92,21.92,31.)) ;
#44327=CARTESIAN_POINT('Origin',(21.92,21.92,49.5)) ;
#44328=CARTESIAN_POINT('',(20.72,21.92,49.5)) ;
#44329=CARTESIAN_POINT('Origin',(-10.5,22.,31.)) ;
#44330=CARTESIAN_POINT('',(-23.42,21.92,31.)) ;
#44331=CARTESIAN_POINT('Origin',(-21.92,21.92,31.)) ;
#44332=CARTESIAN_POINT('Origin',(-21.92,21.92,68.)) ;
#44333=CARTESIAN_POINT('',(-23.42,21.92,68.)) ;
#44334=CARTESIAN_POINT('Origin',(-21.92,21.92,68.)) ;
#44335=CARTESIAN_POINT('',(-23.12,21.92,68.)) ;
#44336=CARTESIAN_POINT('Origin',(-21.92,21.92,68.)) ;
#44337=CARTESIAN_POINT('Origin',(-21.92,21.92,49.5)) ;
#44338=CARTESIAN_POINT('',(-23.42,21.92,49.5)) ;
#44339=CARTESIAN_POINT('Origin',(-21.92,21.92,49.5)) ;
#44340=CARTESIAN_POINT('',(-23.12,21.92,49.5)) ;
#44341=CARTESIAN_POINT('Origin',(-53.,0.,25.)) ;
#44342=CARTESIAN_POINT('',(-55.2360679774998,-24.,27.)) ;
#44343=CARTESIAN_POINT('',(-55.2360679774998,-20.,27.)) ;
#44344=CARTESIAN_POINT('',(-55.2360679774998,0.,27.)) ;
#44345=CARTESIAN_POINT('Origin',(-53.,-20.,25.)) ;
#44346=CARTESIAN_POINT('Origin',(-53.,-24.,25.)) ;
#44347=CARTESIAN_POINT('Origin',(-53.,-24.,25.)) ;
#44348=CARTESIAN_POINT('Origin',(-53.,-24.,43.3)) ;
#44349=CARTESIAN_POINT('',(-31.75,-24.,27.)) ;
#44350=CARTESIAN_POINT('Origin',(-53.,-24.,43.3)) ;
#44351=CARTESIAN_POINT('',(-50.,-24.,43.3)) ;
#44352=CARTESIAN_POINT('Origin',(-53.,-24.,43.3)) ;
#44353=CARTESIAN_POINT('',(-50.,-24.,43.3)) ;
#44354=CARTESIAN_POINT('Origin',(35.,-22.,29.)) ;
#44355=CARTESIAN_POINT('',(35.,-24.,27.)) ;
#44356=CARTESIAN_POINT('',(35.,-24.,29.)) ;
#44357=CARTESIAN_POINT('',(35.,-20.,27.)) ;
#44358=CARTESIAN_POINT('',(35.,-22.,27.)) ;
#44359=CARTESIAN_POINT('',(35.,-20.,29.)) ;
#44360=CARTESIAN_POINT('Origin',(-10.5,-20.,29.)) ;
#44361=CARTESIAN_POINT('',(-10.5,-20.,27.)) ;
#44362=CARTESIAN_POINT('',(-10.5,-20.,27.)) ;
#44363=CARTESIAN_POINT('Origin',(-10.5,-22.,31.)) ;
#44364=CARTESIAN_POINT('Origin',(-10.5,-22.,27.)) ;
#44365=CARTESIAN_POINT('Origin',(-10.5,-22.,27.)) ;
#44366=CARTESIAN_POINT('',(-10.5,-24.,27.)) ;
#44367=CARTESIAN_POINT('Origin',(-10.5,-24.,29.)) ;
#44368=CARTESIAN_POINT('',(-50.,-24.,43.3)) ;
#44369=CARTESIAN_POINT('Origin',(-53.,27.,86.)) ;
#44370=CARTESIAN_POINT('',(-50.,-4.8,86.)) ;
#44371=CARTESIAN_POINT('',(-53.,-4.8,86.)) ;
#44372=CARTESIAN_POINT('',(-50.,27.,86.)) ;
#44373=CARTESIAN_POINT('Origin',(-50.,27.,43.3)) ;
#44374=CARTESIAN_POINT('',(-50.,-4.,82.)) ;
#44375=CARTESIAN_POINT('',(-50.,-4.,65.65)) ;
#44376=CARTESIAN_POINT('',(-50.,-4.8,82.)) ;
#44377=CARTESIAN_POINT('',(-50.,11.3,82.)) ;
#44378=CARTESIAN_POINT('',(-50.,-4.8,65.65)) ;
#44379=CARTESIAN_POINT('Origin',(-49.,-4.4,88.)) ;
#44380=CARTESIAN_POINT('',(-49.,-4.8,94.)) ;
#44381=CARTESIAN_POINT('',(-49.,-4.8,82.)) ;
#44382=CARTESIAN_POINT('',(-49.,-4.8,88.)) ;
#44383=CARTESIAN_POINT('',(-49.,-4.,82.)) ;
#44384=CARTESIAN_POINT('',(-49.,-4.4,82.)) ;
#44385=CARTESIAN_POINT('',(-49.,-4.,94.)) ;
#44386=CARTESIAN_POINT('',(-49.,-4.,88.)) ;
#44387=CARTESIAN_POINT('',(-49.,-4.4,94.)) ;
#44388=CARTESIAN_POINT('Origin',(-57.,-4.4,88.)) ;
#44389=CARTESIAN_POINT('',(-57.,-4.,94.)) ;
#44390=CARTESIAN_POINT('',(-57.,-4.,82.)) ;
#44391=CARTESIAN_POINT('',(-57.,-4.,88.)) ;
#44392=CARTESIAN_POINT('',(-57.,-4.8,82.)) ;
#44393=CARTESIAN_POINT('',(-57.,-4.4,82.)) ;
#44394=CARTESIAN_POINT('',(-57.,-4.8,94.)) ;
#44395=CARTESIAN_POINT('',(-57.,-4.8,88.)) ;
#44396=CARTESIAN_POINT('',(-57.,-4.4,94.)) ;
#44397=CARTESIAN_POINT('Origin',(-53.,-4.8,88.)) ;
#44398=CARTESIAN_POINT('',(-53.,-4.8,82.)) ;
#44399=CARTESIAN_POINT('',(-53.,-4.8,94.)) ;
#44400=CARTESIAN_POINT('',(-53.,-4.8,82.)) ;
#44401=CARTESIAN_POINT('Origin',(-53.,-4.4,82.)) ;
#44402=CARTESIAN_POINT('',(-53.,-4.,82.)) ;
#44403=CARTESIAN_POINT('Origin',(-53.,-4.4,94.)) ;
#44404=CARTESIAN_POINT('',(-53.,-4.,94.)) ;
#44405=CARTESIAN_POINT('Origin',(-53.,-4.,88.)) ;
#44406=CARTESIAN_POINT('',(-53.,-4.,82.)) ;
#44407=CARTESIAN_POINT('Origin',(-53.,-4.4,82.)) ;
#44408=CARTESIAN_POINT('Origin',(-53.,0.,25.)) ;
#44409=CARTESIAN_POINT('',(-50.4,24.4,26.4966629547096)) ;
#44410=CARTESIAN_POINT('',(-55.6,24.4,26.4966629547096)) ;
#44411=CARTESIAN_POINT('Origin',(-53.,24.4,25.)) ;
#44412=CARTESIAN_POINT('',(-50.4,29.6,26.4966629547096)) ;
#44413=CARTESIAN_POINT('',(-50.4,0.,26.4966629547096)) ;
#44414=CARTESIAN_POINT('',(-55.6,29.6,26.4966629547096)) ;
#44415=CARTESIAN_POINT('Origin',(-53.,29.6,25.)) ;
#44416=CARTESIAN_POINT('',(-55.6,0.,26.4966629547096)) ;
#44417=CARTESIAN_POINT('Origin',(-55.6,27.,43.3)) ;
#44418=CARTESIAN_POINT('',(-55.6,29.6,80.)) ;
#44419=CARTESIAN_POINT('',(-55.6,29.6,43.3)) ;
#44420=CARTESIAN_POINT('',(-55.6,24.4,80.)) ;
#44421=CARTESIAN_POINT('',(-55.6,13.5,80.)) ;
#44422=CARTESIAN_POINT('',(-55.6,24.4,43.3)) ;
#44423=CARTESIAN_POINT('Origin',(-53.,29.6,43.3)) ;
#44424=CARTESIAN_POINT('',(-50.4,29.6,80.)) ;
#44425=CARTESIAN_POINT('',(-50.4,29.6,43.3)) ;
#44426=CARTESIAN_POINT('',(-53.,29.6,80.)) ;
#44427=CARTESIAN_POINT('Origin',(-50.4,27.,43.3)) ;
#44428=CARTESIAN_POINT('',(-50.4,24.4,80.)) ;
#44429=CARTESIAN_POINT('',(-50.4,24.4,43.3)) ;
#44430=CARTESIAN_POINT('',(-50.4,13.5,80.)) ;
#44431=CARTESIAN_POINT('Origin',(-53.,24.4,43.3)) ;
#44432=CARTESIAN_POINT('',(-53.,24.4,80.)) ;
#44433=CARTESIAN_POINT('Origin',(-53.,0.,80.)) ;
#44434=CARTESIAN_POINT('Origin',(-53.,0.,80.)) ;
#44435=CARTESIAN_POINT('',(-50.4,-24.4,80.)) ;
#44436=CARTESIAN_POINT('',(-55.6,-24.4,80.)) ;
#44437=CARTESIAN_POINT('',(-53.,-24.4,80.)) ;
#44438=CARTESIAN_POINT('',(-50.4,-29.6,80.)) ;
#44439=CARTESIAN_POINT('',(-50.4,-13.5,80.)) ;
#44440=CARTESIAN_POINT('',(-55.6,-29.6,80.)) ;
#44441=CARTESIAN_POINT('',(-53.,-29.6,80.)) ;
#44442=CARTESIAN_POINT('',(-55.6,-13.5,80.)) ;
#44443=CARTESIAN_POINT('Origin',(-53.,-29.6,43.3)) ;
#44444=CARTESIAN_POINT('',(-50.4,-29.6,26.4966629547096)) ;
#44445=CARTESIAN_POINT('',(-55.6,-29.6,26.4966629547096)) ;
#44446=CARTESIAN_POINT('Origin',(-53.,-29.6,25.)) ;
#44447=CARTESIAN_POINT('',(-55.6,-29.6,43.3)) ;
#44448=CARTESIAN_POINT('',(-50.4,-29.6,43.3)) ;
#44449=CARTESIAN_POINT('Origin',(-50.4,-27.,43.3)) ;
#44450=CARTESIAN_POINT('',(-50.4,-24.4,26.4966629547096)) ;
#44451=CARTESIAN_POINT('',(-50.4,0.,26.4966629547096)) ;
#44452=CARTESIAN_POINT('',(-50.4,-24.4,43.3)) ;
#44453=CARTESIAN_POINT('Origin',(-53.,-24.4,43.3)) ;
#44454=CARTESIAN_POINT('',(-55.6,-24.4,26.4966629547096)) ;
#44455=CARTESIAN_POINT('Origin',(-53.,-24.4,25.)) ;
#44456=CARTESIAN_POINT('',(-55.6,-24.4,43.3)) ;
#44457=CARTESIAN_POINT('Origin',(-55.6,-27.,43.3)) ;
#44458=CARTESIAN_POINT('',(-55.6,0.,26.4966629547096)) ;
#44459=CARTESIAN_POINT('Origin',(-53.,0.,25.)) ;
#44460=CARTESIAN_POINT('Origin',(-10.5,23.6,29.)) ;
#44461=CARTESIAN_POINT('',(-54.5329709716756,23.6,27.1)) ;
#44462=CARTESIAN_POINT('',(-51.4670290283244,23.6,27.1)) ;
#44463=CARTESIAN_POINT('Origin',(-53.,23.6,25.)) ;
#44464=CARTESIAN_POINT('',(-10.5,23.6,27.1)) ;
#44465=CARTESIAN_POINT('Origin',(-10.5,20.4,29.)) ;
#44466=CARTESIAN_POINT('',(-51.4670290283244,20.4,27.1)) ;
#44467=CARTESIAN_POINT('',(-54.5329709716756,20.4,27.1)) ;
#44468=CARTESIAN_POINT('Origin',(-53.,20.4,25.)) ;
#44469=CARTESIAN_POINT('',(-10.5,20.4,27.1)) ;
#44470=CARTESIAN_POINT('Origin',(-10.5,22.,27.1)) ;
#44471=CARTESIAN_POINT('',(-51.4670290283244,0.,27.1)) ;
#44472=CARTESIAN_POINT('',(-54.5329709716756,0.,27.1)) ;
#44473=CARTESIAN_POINT('Origin',(-53.,0.,25.)) ;
#44474=CARTESIAN_POINT('Origin',(-53.,0.,22.4)) ;
#44475=CARTESIAN_POINT('',(-51.5033370452904,24.,22.4)) ;
#44476=CARTESIAN_POINT('',(-50.4,24.,22.4)) ;
#44477=CARTESIAN_POINT('',(-53.,24.,22.4)) ;
#44478=CARTESIAN_POINT('',(-51.5033370452904,-24.,22.4)) ;
#44479=CARTESIAN_POINT('',(-51.5033370452904,0.,22.4)) ;
#44480=CARTESIAN_POINT('',(-50.4,-24.,22.4)) ;
#44481=CARTESIAN_POINT('',(-53.,-24.,22.4)) ;
#44482=CARTESIAN_POINT('',(-50.4,0.,22.4)) ;
#44483=CARTESIAN_POINT('Origin',(-50.4,0.,24.)) ;
#44484=CARTESIAN_POINT('',(-50.4,24.,23.5033370452904)) ;
#44485=CARTESIAN_POINT('',(-50.4,24.,33.65)) ;
#44486=CARTESIAN_POINT('',(-50.4,-24.,23.5033370452904)) ;
#44487=CARTESIAN_POINT('',(-50.4,-24.,33.65)) ;
#44488=CARTESIAN_POINT('',(-50.4,0.,23.5033370452904)) ;
#44489=CARTESIAN_POINT('Origin',(-53.,24.,43.3)) ;
#44490=CARTESIAN_POINT('Origin',(-53.,24.,25.)) ;
#44491=CARTESIAN_POINT('Origin',(-53.,-24.,43.3)) ;
#44492=CARTESIAN_POINT('Origin',(-53.,-24.,25.)) ;
#44493=CARTESIAN_POINT('Origin',(-53.,0.,25.)) ;
#44494=CARTESIAN_POINT('Origin',(-53.,29.6,43.3)) ;
#44495=CARTESIAN_POINT('',(-55.6,29.6,22.4)) ;
#44496=CARTESIAN_POINT('',(-54.4966629547096,29.6,22.4)) ;
#44497=CARTESIAN_POINT('',(-53.,29.6,22.4)) ;
#44498=CARTESIAN_POINT('',(-55.6,29.6,23.5033370452904)) ;
#44499=CARTESIAN_POINT('Origin',(-53.,29.6,25.)) ;
#44500=CARTESIAN_POINT('',(-55.6,29.6,43.3)) ;
#44501=CARTESIAN_POINT('Origin',(-55.6,27.,43.3)) ;
#44502=CARTESIAN_POINT('',(-55.6,24.4,22.4)) ;
#44503=CARTESIAN_POINT('',(-55.6,13.5,22.4)) ;
#44504=CARTESIAN_POINT('',(-55.6,24.4,23.5033370452904)) ;
#44505=CARTESIAN_POINT('',(-55.6,0.,23.5033370452904)) ;
#44506=CARTESIAN_POINT('',(-55.6,24.4,43.3)) ;
#44507=CARTESIAN_POINT('Origin',(-53.,24.4,43.3)) ;
#44508=CARTESIAN_POINT('',(-54.4966629547096,24.4,22.4)) ;
#44509=CARTESIAN_POINT('',(-53.,24.4,22.4)) ;
#44510=CARTESIAN_POINT('Origin',(-53.,24.4,25.)) ;
#44511=CARTESIAN_POINT('Origin',(-53.,0.,25.)) ;
#44512=CARTESIAN_POINT('',(-54.4966629547096,0.,22.4)) ;
#44513=CARTESIAN_POINT('Origin',(-53.,0.,22.4)) ;
#44514=CARTESIAN_POINT('Origin',(-53.,0.,22.4)) ;
#44515=CARTESIAN_POINT('',(-55.6,24.,22.4)) ;
#44516=CARTESIAN_POINT('',(-54.4966629547096,24.,22.4)) ;
#44517=CARTESIAN_POINT('',(-53.,24.,22.4)) ;
#44518=CARTESIAN_POINT('',(-55.6,-24.,22.4)) ;
#44519=CARTESIAN_POINT('',(-55.6,0.,22.4)) ;
#44520=CARTESIAN_POINT('',(-54.4966629547096,-24.,22.4)) ;
#44521=CARTESIAN_POINT('',(-53.,-24.,22.4)) ;
#44522=CARTESIAN_POINT('',(-54.4966629547096,0.,22.4)) ;
#44523=CARTESIAN_POINT('Origin',(-55.6,0.,24.)) ;
#44524=CARTESIAN_POINT('',(-55.6,24.,23.5033370452904)) ;
#44525=CARTESIAN_POINT('',(-55.6,24.,33.65)) ;
#44526=CARTESIAN_POINT('',(-55.6,-24.,23.5033370452904)) ;
#44527=CARTESIAN_POINT('',(-55.6,0.,23.5033370452904)) ;
#44528=CARTESIAN_POINT('',(-55.6,-24.,33.65)) ;
#44529=CARTESIAN_POINT('Origin',(-53.,24.,43.3)) ;
#44530=CARTESIAN_POINT('Origin',(-53.,24.,25.)) ;
#44531=CARTESIAN_POINT('Origin',(-53.,-24.,43.3)) ;
#44532=CARTESIAN_POINT('Origin',(-53.,-24.,25.)) ;
#44533=CARTESIAN_POINT('Origin',(-53.,0.,25.)) ;
#44534=CARTESIAN_POINT('Origin',(-53.,29.6,43.3)) ;
#44535=CARTESIAN_POINT('',(-51.5033370452904,29.6,22.4)) ;
#44536=CARTESIAN_POINT('',(-50.4,29.6,22.4)) ;
#44537=CARTESIAN_POINT('',(-53.,29.6,22.4)) ;
#44538=CARTESIAN_POINT('',(-50.4,29.6,23.5033370452904)) ;
#44539=CARTESIAN_POINT('',(-50.4,29.6,43.3)) ;
#44540=CARTESIAN_POINT('Origin',(-53.,29.6,25.)) ;
#44541=CARTESIAN_POINT('Origin',(-53.,24.4,43.3)) ;
#44542=CARTESIAN_POINT('',(-50.4,24.4,22.4)) ;
#44543=CARTESIAN_POINT('',(-51.5033370452904,24.4,22.4)) ;
#44544=CARTESIAN_POINT('',(-53.,24.4,22.4)) ;
#44545=CARTESIAN_POINT('',(-50.4,24.4,23.5033370452904)) ;
#44546=CARTESIAN_POINT('Origin',(-53.,24.4,25.)) ;
#44547=CARTESIAN_POINT('',(-50.4,24.4,43.3)) ;
#44548=CARTESIAN_POINT('Origin',(-53.,0.,25.)) ;
#44549=CARTESIAN_POINT('',(-51.5033370452904,0.,22.4)) ;
#44550=CARTESIAN_POINT('',(-50.4,0.,23.5033370452904)) ;
#44551=CARTESIAN_POINT('Origin',(-50.4,27.,43.3)) ;
#44552=CARTESIAN_POINT('',(-50.4,13.5,22.4)) ;
#44553=CARTESIAN_POINT('Origin',(-53.,0.,22.4)) ;
#44554=CARTESIAN_POINT('Origin',(-53.,0.,22.4)) ;
#44555=CARTESIAN_POINT('',(-54.4966629547096,-29.6,22.4)) ;
#44556=CARTESIAN_POINT('',(-55.6,-29.6,22.4)) ;
#44557=CARTESIAN_POINT('',(-53.,-29.6,22.4)) ;
#44558=CARTESIAN_POINT('',(-54.4966629547096,-24.4,22.4)) ;
#44559=CARTESIAN_POINT('',(-54.4966629547096,0.,22.4)) ;
#44560=CARTESIAN_POINT('',(-55.6,-24.4,22.4)) ;
#44561=CARTESIAN_POINT('',(-53.,-24.4,22.4)) ;
#44562=CARTESIAN_POINT('',(-55.6,-13.5,22.4)) ;
#44563=CARTESIAN_POINT('Origin',(-53.,0.,25.)) ;
#44564=CARTESIAN_POINT('',(-55.6,-29.6,23.5033370452904)) ;
#44565=CARTESIAN_POINT('Origin',(-53.,-29.6,25.)) ;
#44566=CARTESIAN_POINT('',(-55.6,-24.4,23.5033370452904)) ;
#44567=CARTESIAN_POINT('',(-55.6,0.,23.5033370452904)) ;
#44568=CARTESIAN_POINT('Origin',(-53.,-24.4,25.)) ;
#44569=CARTESIAN_POINT('Origin',(-53.,-29.6,43.3)) ;
#44570=CARTESIAN_POINT('',(-55.6,-29.6,43.3)) ;
#44571=CARTESIAN_POINT('Origin',(-55.6,-27.,43.3)) ;
#44572=CARTESIAN_POINT('',(-55.6,-24.4,43.3)) ;
#44573=CARTESIAN_POINT('Origin',(-53.,-24.4,43.3)) ;
#44574=CARTESIAN_POINT('Origin',(-53.,-24.4,43.3)) ;
#44575=CARTESIAN_POINT('',(-51.5033370452904,-24.4,22.4)) ;
#44576=CARTESIAN_POINT('',(-50.4,-24.4,22.4)) ;
#44577=CARTESIAN_POINT('',(-53.,-24.4,22.4)) ;
#44578=CARTESIAN_POINT('',(-50.4,-24.4,23.5033370452904)) ;
#44579=CARTESIAN_POINT('',(-50.4,-24.4,43.3)) ;
#44580=CARTESIAN_POINT('Origin',(-53.,-24.4,25.)) ;
#44581=CARTESIAN_POINT('Origin',(-53.,-29.6,43.3)) ;
#44582=CARTESIAN_POINT('',(-50.4,-29.6,22.4)) ;
#44583=CARTESIAN_POINT('',(-51.5033370452904,-29.6,22.4)) ;
#44584=CARTESIAN_POINT('',(-53.,-29.6,22.4)) ;
#44585=CARTESIAN_POINT('',(-50.4,-29.6,23.5033370452904)) ;
#44586=CARTESIAN_POINT('Origin',(-53.,-29.6,25.)) ;
#44587=CARTESIAN_POINT('',(-50.4,-29.6,43.3)) ;
#44588=CARTESIAN_POINT('Origin',(-53.,0.,25.)) ;
#44589=CARTESIAN_POINT('',(-51.5033370452904,0.,22.4)) ;
#44590=CARTESIAN_POINT('',(-50.4,0.,23.5033370452904)) ;
#44591=CARTESIAN_POINT('Origin',(-50.4,-27.,43.3)) ;
#44592=CARTESIAN_POINT('',(-50.4,-13.5,22.4)) ;
#44593=CARTESIAN_POINT('Origin',(-53.,0.,22.4)) ;
#44594=CARTESIAN_POINT('Origin',(-53.,0.,25.6)) ;
#44595=CARTESIAN_POINT('',(-55.5298221281347,29.6,25.6)) ;
#44596=CARTESIAN_POINT('',(-55.5298221281347,24.4,25.6)) ;
#44597=CARTESIAN_POINT('',(-55.5298221281347,0.,25.6)) ;
#44598=CARTESIAN_POINT('',(-50.4701778718653,29.6,25.6)) ;
#44599=CARTESIAN_POINT('',(-53.,29.6,25.6)) ;
#44600=CARTESIAN_POINT('',(-50.4701778718653,24.4,25.6)) ;
#44601=CARTESIAN_POINT('',(-50.4701778718653,0.,25.6)) ;
#44602=CARTESIAN_POINT('',(-53.,24.4,25.6)) ;
#44603=CARTESIAN_POINT('Origin',(-53.,24.4,43.3)) ;
#44604=CARTESIAN_POINT('Origin',(-53.,24.4,25.)) ;
#44605=CARTESIAN_POINT('Origin',(-53.,29.6,43.3)) ;
#44606=CARTESIAN_POINT('Origin',(-53.,29.6,25.)) ;
#44607=CARTESIAN_POINT('Origin',(-53.,0.,25.)) ;
#44608=CARTESIAN_POINT('Origin',(-53.,0.,25.)) ;
#44609=CARTESIAN_POINT('',(-50.4701778718653,-29.6,25.6)) ;
#44610=CARTESIAN_POINT('',(-50.4701778718653,-24.4,25.6)) ;
#44611=CARTESIAN_POINT('',(-50.4701778718653,0.,25.6)) ;
#44612=CARTESIAN_POINT('',(-55.5298221281347,-24.4,25.6)) ;
#44613=CARTESIAN_POINT('Origin',(-53.,-24.4,25.)) ;
#44614=CARTESIAN_POINT('',(-55.5298221281347,-29.6,25.6)) ;
#44615=CARTESIAN_POINT('',(-55.5298221281347,0.,25.6)) ;
#44616=CARTESIAN_POINT('Origin',(-53.,-29.6,25.)) ;
#44617=CARTESIAN_POINT('Origin',(-53.,-29.6,43.3)) ;
#44618=CARTESIAN_POINT('',(-53.,-29.6,25.6)) ;
#44619=CARTESIAN_POINT('Origin',(-53.,-24.4,43.3)) ;
#44620=CARTESIAN_POINT('',(-53.,-24.4,25.6)) ;
#44621=CARTESIAN_POINT('Origin',(-53.,0.,25.6)) ;
#44622=CARTESIAN_POINT('Origin',(-53.,0.,26.)) ;
#44623=CARTESIAN_POINT('',(-50.6,-29.6,26.)) ;
#44624=CARTESIAN_POINT('',(-55.4,-29.6,26.)) ;
#44625=CARTESIAN_POINT('',(-53.,-29.6,26.)) ;
#44626=CARTESIAN_POINT('',(-50.6,-24.4,26.)) ;
#44627=CARTESIAN_POINT('',(-50.6,0.,26.)) ;
#44628=CARTESIAN_POINT('',(-55.4,-24.4,26.)) ;
#44629=CARTESIAN_POINT('',(-53.,-24.4,26.)) ;
#44630=CARTESIAN_POINT('',(-55.4,0.,26.)) ;
#44631=CARTESIAN_POINT('Origin',(-53.,-24.4,43.3)) ;
#44632=CARTESIAN_POINT('Origin',(-53.,-24.4,25.)) ;
#44633=CARTESIAN_POINT('Origin',(-53.,-29.6,43.3)) ;
#44634=CARTESIAN_POINT('Origin',(-53.,-29.6,25.)) ;
#44635=CARTESIAN_POINT('Origin',(-53.,0.,25.)) ;
#44636=CARTESIAN_POINT('Origin',(-53.,0.,25.)) ;
#44637=CARTESIAN_POINT('',(-50.4701778718653,-24.,25.6)) ;
#44638=CARTESIAN_POINT('',(-50.4701778718653,24.,25.6)) ;
#44639=CARTESIAN_POINT('',(-50.4701778718653,0.,25.6)) ;
#44640=CARTESIAN_POINT('',(-55.5298221281347,24.,25.6)) ;
#44641=CARTESIAN_POINT('Origin',(-53.,24.,25.)) ;
#44642=CARTESIAN_POINT('',(-55.5298221281347,-24.,25.6)) ;
#44643=CARTESIAN_POINT('',(-55.5298221281347,0.,25.6)) ;
#44644=CARTESIAN_POINT('Origin',(-53.,-24.,25.)) ;
#44645=CARTESIAN_POINT('Origin',(-53.,24.,43.3)) ;
#44646=CARTESIAN_POINT('',(-53.,24.,25.6)) ;
#44647=CARTESIAN_POINT('Origin',(-53.,-24.,43.3)) ;
#44648=CARTESIAN_POINT('',(-53.,-24.,25.6)) ;
#44649=CARTESIAN_POINT('Origin',(-53.,0.,25.6)) ;
#44650=CARTESIAN_POINT('Origin',(-53.,0.,26.)) ;
#44651=CARTESIAN_POINT('',(-55.4,24.4,26.)) ;
#44652=CARTESIAN_POINT('',(-55.4,29.6,26.)) ;
#44653=CARTESIAN_POINT('',(-55.4,0.,26.)) ;
#44654=CARTESIAN_POINT('',(-50.6,24.4,26.)) ;
#44655=CARTESIAN_POINT('',(-53.,24.4,26.)) ;
#44656=CARTESIAN_POINT('',(-50.6,29.6,26.)) ;
#44657=CARTESIAN_POINT('',(-50.6,0.,26.)) ;
#44658=CARTESIAN_POINT('',(-53.,29.6,26.)) ;
#44659=CARTESIAN_POINT('Origin',(-53.,24.4,43.3)) ;
#44660=CARTESIAN_POINT('Origin',(-53.,24.4,25.)) ;
#44661=CARTESIAN_POINT('Origin',(-53.,0.,25.)) ;
#44662=CARTESIAN_POINT('Origin',(-53.,29.6,25.)) ;
#44663=CARTESIAN_POINT('Origin',(-53.,29.6,43.3)) ;
#44664=CARTESIAN_POINT('Origin',(-53.,29.6,43.3)) ;
#44665=CARTESIAN_POINT('',(-50.4,29.6,85.6)) ;
#44666=CARTESIAN_POINT('',(-55.6,29.6,85.6)) ;
#44667=CARTESIAN_POINT('',(-53.,29.6,85.6)) ;
#44668=CARTESIAN_POINT('',(-55.6,29.6,80.4)) ;
#44669=CARTESIAN_POINT('',(-55.6,29.6,43.3)) ;
#44670=CARTESIAN_POINT('',(-50.4,29.6,80.4)) ;
#44671=CARTESIAN_POINT('',(-53.,29.6,80.4)) ;
#44672=CARTESIAN_POINT('',(-50.4,29.6,43.3)) ;
#44673=CARTESIAN_POINT('Origin',(-55.6,27.,43.3)) ;
#44674=CARTESIAN_POINT('',(-55.6,24.4,85.6)) ;
#44675=CARTESIAN_POINT('',(-55.6,13.5,85.6)) ;
#44676=CARTESIAN_POINT('',(-55.6,24.4,80.4)) ;
#44677=CARTESIAN_POINT('',(-55.6,24.4,43.3)) ;
#44678=CARTESIAN_POINT('',(-55.6,13.5,80.4)) ;
#44679=CARTESIAN_POINT('Origin',(-50.4,27.,43.3)) ;
#44680=CARTESIAN_POINT('',(-50.4,24.4,85.6)) ;
#44681=CARTESIAN_POINT('',(-50.4,13.5,85.6)) ;
#44682=CARTESIAN_POINT('',(-50.4,24.4,80.4)) ;
#44683=CARTESIAN_POINT('',(-50.4,13.5,80.4)) ;
#44684=CARTESIAN_POINT('',(-50.4,24.4,43.3)) ;
#44685=CARTESIAN_POINT('Origin',(-53.,24.4,43.3)) ;
#44686=CARTESIAN_POINT('',(-53.,24.4,85.6)) ;
#44687=CARTESIAN_POINT('',(-53.,24.4,80.4)) ;
#44688=CARTESIAN_POINT('Origin',(-53.,0.,80.4)) ;
#44689=CARTESIAN_POINT('Origin',(-53.,0.,85.6)) ;
#44690=CARTESIAN_POINT('Origin',(-53.,0.,85.6)) ;
#44691=CARTESIAN_POINT('',(-55.6,-29.6,85.6)) ;
#44692=CARTESIAN_POINT('',(-50.4,-29.6,85.6)) ;
#44693=CARTESIAN_POINT('',(-53.,-29.6,85.6)) ;
#44694=CARTESIAN_POINT('',(-55.6,-24.4,85.6)) ;
#44695=CARTESIAN_POINT('',(-55.6,-13.5,85.6)) ;
#44696=CARTESIAN_POINT('',(-50.4,-24.4,85.6)) ;
#44697=CARTESIAN_POINT('',(-53.,-24.4,85.6)) ;
#44698=CARTESIAN_POINT('',(-50.4,-13.5,85.6)) ;
#44699=CARTESIAN_POINT('Origin',(-53.,0.,80.4)) ;
#44700=CARTESIAN_POINT('',(-50.4,-29.6,80.4)) ;
#44701=CARTESIAN_POINT('',(-55.6,-29.6,80.4)) ;
#44702=CARTESIAN_POINT('',(-53.,-29.6,80.4)) ;
#44703=CARTESIAN_POINT('',(-50.4,-24.4,80.4)) ;
#44704=CARTESIAN_POINT('',(-50.4,-13.5,80.4)) ;
#44705=CARTESIAN_POINT('',(-55.6,-24.4,80.4)) ;
#44706=CARTESIAN_POINT('',(-53.,-24.4,80.4)) ;
#44707=CARTESIAN_POINT('',(-55.6,-13.5,80.4)) ;
#44708=CARTESIAN_POINT('Origin',(-53.,-29.6,43.3)) ;
#44709=CARTESIAN_POINT('',(-50.4,-29.6,43.3)) ;
#44710=CARTESIAN_POINT('',(-55.6,-29.6,43.3)) ;
#44711=CARTESIAN_POINT('Origin',(-50.4,-27.,43.3)) ;
#44712=CARTESIAN_POINT('',(-50.4,-24.4,43.3)) ;
#44713=CARTESIAN_POINT('Origin',(-55.6,-27.,43.3)) ;
#44714=CARTESIAN_POINT('',(-55.6,-24.4,43.3)) ;
#44715=CARTESIAN_POINT('Origin',(-53.,-24.4,43.3)) ;
#44716=CARTESIAN_POINT('Origin',(-53.,-4.8,88.)) ;
#44717=CARTESIAN_POINT('',(-55.6,-4.8,82.)) ;
#44718=CARTESIAN_POINT('',(-55.6,-4.8,85.6)) ;
#44719=CARTESIAN_POINT('',(-55.6,-4.8,85.5)) ;
#44720=CARTESIAN_POINT('',(-50.4,-4.8,82.)) ;
#44721=CARTESIAN_POINT('',(-53.,-4.8,82.)) ;
#44722=CARTESIAN_POINT('',(-50.4,-4.8,85.6)) ;
#44723=CARTESIAN_POINT('',(-50.4,-4.8,85.5)) ;
#44724=CARTESIAN_POINT('',(-53.,-4.8,85.6)) ;
#44725=CARTESIAN_POINT('Origin',(-53.,-4.4,82.)) ;
#44726=CARTESIAN_POINT('',(-55.6,-4.,82.)) ;
#44727=CARTESIAN_POINT('',(-55.6,-2.2,82.)) ;
#44728=CARTESIAN_POINT('',(-50.4,-4.,82.)) ;
#44729=CARTESIAN_POINT('',(-53.,-4.,82.)) ;
#44730=CARTESIAN_POINT('',(-50.4,-2.2,82.)) ;
#44731=CARTESIAN_POINT('Origin',(-53.,-4.,88.)) ;
#44732=CARTESIAN_POINT('',(-55.6,-4.,85.6)) ;
#44733=CARTESIAN_POINT('',(-55.6,-4.,85.5)) ;
#44734=CARTESIAN_POINT('',(-50.4,-4.,85.6)) ;
#44735=CARTESIAN_POINT('',(-53.,-4.,85.6)) ;
#44736=CARTESIAN_POINT('',(-50.4,-4.,85.5)) ;
#44737=CARTESIAN_POINT('Origin',(-50.4,0.,83.)) ;
#44738=CARTESIAN_POINT('',(-50.4,4.,85.6)) ;
#44739=CARTESIAN_POINT('',(-50.4,0.,85.6)) ;
#44740=CARTESIAN_POINT('',(-50.4,4.,82.)) ;
#44741=CARTESIAN_POINT('',(-50.4,4.,85.5)) ;
#44742=CARTESIAN_POINT('',(-50.4,4.8,82.)) ;
#44743=CARTESIAN_POINT('',(-50.4,2.2,82.)) ;
#44744=CARTESIAN_POINT('',(-50.4,4.8,85.6)) ;
#44745=CARTESIAN_POINT('',(-50.4,4.8,85.5)) ;
#44746=CARTESIAN_POINT('',(-50.4,24.,85.6)) ;
#44747=CARTESIAN_POINT('',(-50.4,0.,85.6)) ;
#44748=CARTESIAN_POINT('',(-50.4,24.,80.4)) ;
#44749=CARTESIAN_POINT('',(-50.4,24.,63.15)) ;
#44750=CARTESIAN_POINT('',(-50.4,-24.,80.4)) ;
#44751=CARTESIAN_POINT('',(-50.4,0.,80.4)) ;
#44752=CARTESIAN_POINT('',(-50.4,-24.,85.6)) ;
#44753=CARTESIAN_POINT('',(-50.4,-24.,63.15)) ;
#44754=CARTESIAN_POINT('',(-50.4,0.,85.6)) ;
#44755=CARTESIAN_POINT('Origin',(-53.,0.,85.6)) ;
#44756=CARTESIAN_POINT('',(-55.6,4.,85.6)) ;
#44757=CARTESIAN_POINT('',(-55.6,0.,85.6)) ;
#44758=CARTESIAN_POINT('',(-53.,4.,85.6)) ;
#44759=CARTESIAN_POINT('Origin',(-53.,0.,85.6)) ;
#44760=CARTESIAN_POINT('',(-55.6,-24.,85.6)) ;
#44761=CARTESIAN_POINT('',(-53.,-24.,85.6)) ;
#44762=CARTESIAN_POINT('',(-55.6,0.,85.6)) ;
#44763=CARTESIAN_POINT('Origin',(-55.6,0.,83.)) ;
#44764=CARTESIAN_POINT('',(-55.6,-24.,80.4)) ;
#44765=CARTESIAN_POINT('',(-55.6,-24.,63.15)) ;
#44766=CARTESIAN_POINT('',(-55.6,24.,80.4)) ;
#44767=CARTESIAN_POINT('',(-55.6,0.,80.4)) ;
#44768=CARTESIAN_POINT('',(-55.6,24.,85.6)) ;
#44769=CARTESIAN_POINT('',(-55.6,24.,63.15)) ;
#44770=CARTESIAN_POINT('',(-55.6,4.8,85.6)) ;
#44771=CARTESIAN_POINT('',(-55.6,0.,85.6)) ;
#44772=CARTESIAN_POINT('',(-55.6,4.8,82.)) ;
#44773=CARTESIAN_POINT('',(-55.6,4.8,85.5)) ;
#44774=CARTESIAN_POINT('',(-55.6,4.,82.)) ;
#44775=CARTESIAN_POINT('',(-55.6,2.2,82.)) ;
#44776=CARTESIAN_POINT('',(-55.6,4.,85.5)) ;
#44777=CARTESIAN_POINT('Origin',(-53.,0.,80.4)) ;
#44778=CARTESIAN_POINT('',(-53.,24.,80.4)) ;
#44779=CARTESIAN_POINT('',(-53.,-24.,80.4)) ;
#44780=CARTESIAN_POINT('Origin',(-53.,-24.,43.3)) ;
#44781=CARTESIAN_POINT('Origin',(-53.,24.,43.3)) ;
#44782=CARTESIAN_POINT('',(-53.,24.,85.6)) ;
#44783=CARTESIAN_POINT('Origin',(-53.,0.,85.6)) ;
#44784=CARTESIAN_POINT('',(-53.,4.8,85.6)) ;
#44785=CARTESIAN_POINT('Origin',(-53.,4.8,88.)) ;
#44786=CARTESIAN_POINT('',(-53.,4.8,82.)) ;
#44787=CARTESIAN_POINT('Origin',(-53.,4.4,82.)) ;
#44788=CARTESIAN_POINT('',(-53.,4.,82.)) ;
#44789=CARTESIAN_POINT('Origin',(-53.,4.,88.)) ;
#44790=CARTESIAN_POINT('Origin',(-53.,0.,25.)) ;
#44791=CARTESIAN_POINT('',(-54.5329709716756,-23.6,27.1)) ;
#44792=CARTESIAN_POINT('',(-54.5329709716756,-20.4,27.1)) ;
#44793=CARTESIAN_POINT('',(-54.5329709716756,0.,27.1)) ;
#44794=CARTESIAN_POINT('',(-51.4670290283244,-20.4,27.1)) ;
#44795=CARTESIAN_POINT('Origin',(-53.,-20.4,25.)) ;
#44796=CARTESIAN_POINT('',(-51.4670290283244,-23.6,27.1)) ;
#44797=CARTESIAN_POINT('',(-51.4670290283244,0.,27.1)) ;
#44798=CARTESIAN_POINT('Origin',(-53.,-23.6,25.)) ;
#44799=CARTESIAN_POINT('Origin',(-10.5,-22.,27.1)) ;
#44800=CARTESIAN_POINT('',(-10.5,-20.4,27.1)) ;
#44801=CARTESIAN_POINT('',(-10.5,-23.6,27.1)) ;
#44802=CARTESIAN_POINT('Origin',(-10.5,-23.6,29.)) ;
#44803=CARTESIAN_POINT('Origin',(-10.5,-20.4,29.)) ;
#44804=CARTESIAN_POINT('Origin',(-10.5,-20.,29.)) ;
#44805=CARTESIAN_POINT('',(-51.3386752274164,-20.,27.)) ;
#44806=CARTESIAN_POINT('',(-54.6613247725836,-20.,27.)) ;
#44807=CARTESIAN_POINT('Origin',(-53.,-20.,25.)) ;
#44808=CARTESIAN_POINT('',(-10.5,-20.,27.)) ;
#44809=CARTESIAN_POINT('Origin',(-10.5,-22.,27.)) ;
#44810=CARTESIAN_POINT('',(-51.3386752274164,-24.,27.)) ;
#44811=CARTESIAN_POINT('',(-51.3386752274164,0.,27.)) ;
#44812=CARTESIAN_POINT('',(-54.6613247725836,-24.,27.)) ;
#44813=CARTESIAN_POINT('',(-31.75,-24.,27.)) ;
#44814=CARTESIAN_POINT('',(-54.6613247725836,0.,27.)) ;
#44815=CARTESIAN_POINT('Origin',(-53.,0.,25.)) ;
#44816=CARTESIAN_POINT('',(-55.4,-24.,26.)) ;
#44817=CARTESIAN_POINT('Origin',(-53.,-24.,25.)) ;
#44818=CARTESIAN_POINT('',(-55.4,24.,26.)) ;
#44819=CARTESIAN_POINT('',(-55.4,0.,26.)) ;
#44820=CARTESIAN_POINT('',(-54.6613247725836,24.,27.)) ;
#44821=CARTESIAN_POINT('Origin',(-53.,24.,25.)) ;
#44822=CARTESIAN_POINT('',(-54.6613247725836,20.,27.)) ;
#44823=CARTESIAN_POINT('',(-54.6613247725836,0.,27.)) ;
#44824=CARTESIAN_POINT('',(-51.3386752274164,20.,27.)) ;
#44825=CARTESIAN_POINT('Origin',(-53.,20.,25.)) ;
#44826=CARTESIAN_POINT('',(-51.3386752274164,24.,27.)) ;
#44827=CARTESIAN_POINT('',(-51.3386752274164,0.,27.)) ;
#44828=CARTESIAN_POINT('',(-50.6,24.,26.)) ;
#44829=CARTESIAN_POINT('Origin',(-53.,24.,25.)) ;
#44830=CARTESIAN_POINT('',(-50.6,-24.,26.)) ;
#44831=CARTESIAN_POINT('',(-50.6,0.,26.)) ;
#44832=CARTESIAN_POINT('Origin',(-53.,-24.,25.)) ;
#44833=CARTESIAN_POINT('Origin',(-10.5,20.,29.)) ;
#44834=CARTESIAN_POINT('',(-10.5,20.,27.)) ;
#44835=CARTESIAN_POINT('Origin',(-10.5,22.,27.)) ;
#44836=CARTESIAN_POINT('',(-31.75,24.,27.)) ;
#44837=CARTESIAN_POINT('Origin',(-53.,24.,43.3)) ;
#44838=CARTESIAN_POINT('',(-53.,24.,26.)) ;
#44839=CARTESIAN_POINT('Origin',(-53.,-24.,43.3)) ;
#44840=CARTESIAN_POINT('',(-53.,-24.,26.)) ;
#44841=CARTESIAN_POINT('Origin',(-53.,0.,26.)) ;
#50343=UNCERTAINTY_MEASURE_WITH_UNIT(LENGTH_MEASURE(0.001),#50441,
'DISTANCE_ACCURACY_VALUE',
'Maximum model space distance between geometric entities at asserted c
onnectivities') ;
#50387=UNCERTAINTY_MEASURE_WITH_UNIT(LENGTH_MEASURE(0.001),#50441,
'DISTANCE_ACCURACY_VALUE',
'Maximum model space distance between geometric entities at asserted c
onnectivities') ;
#50396=(
GEOMETRIC_REPRESENTATION_CONTEXT(3)
GLOBAL_UNCERTAINTY_ASSIGNED_CONTEXT((#50343))
GLOBAL_UNIT_ASSIGNED_CONTEXT((#50441,#50443,#50444))
REPRESENTATION_CONTEXT('','3D')
) ;
#50440=(
GEOMETRIC_REPRESENTATION_CONTEXT(3)
GLOBAL_UNCERTAINTY_ASSIGNED_CONTEXT((#50387))
GLOBAL_UNIT_ASSIGNED_CONTEXT((#50441,#50443,#50444))
REPRESENTATION_CONTEXT('','3D')
) ;
#50441=(
LENGTH_UNIT()
NAMED_UNIT(*)
SI_UNIT(.CENTI.,.METRE.)
) ;
#50443=(
NAMED_UNIT(*)
PLANE_ANGLE_UNIT()
SI_UNIT($,.RADIAN.)
) ;
#50444=(
NAMED_UNIT(*)
SI_UNIT($,.STERADIAN.)
SOLID_ANGLE_UNIT()
) ;
#50453=SHAPE_DEFINITION_REPRESENTATION(#50511,#50627) ;
#50511=PRODUCT_DEFINITION_SHAPE('',$,#50680) ;
#50627=SHAPE_REPRESENTATION('',(#29921),#50396) ;
#50671=PRODUCT_DEFINITION_CONTEXT('part definition',#50829,'design') ;
#50680=PRODUCT_DEFINITION('TUBULAR_3POINT_HITCH_FRAME',
'TUBULAR_3POINT_HITCH_FRAME',#50732,#50671) ;
#50732=PRODUCT_DEFINITION_FORMATION('',$,#50839) ;
#50829=APPLICATION_CONTEXT(
'Core Data for Automotive Mechanical Design Process') ;
#50830=PRODUCT_CONTEXT('part definition',#50829,'mechanical') ;
#50839=PRODUCT('TUBULAR_3POINT_HITCH_FRAME','TUBULAR_3POINT_HITCH_FRAME',$,
(#50830)) ;
#50883=PRESENTATION_STYLE_ASSIGNMENT((#50890)) ;
#50890=SURFACE_STYLE_USAGE(.BOTH.,#50897) ;
#50897=SURFACE_SIDE_STYLE('',(#50904)) ;
#50904=SURFACE_STYLE_FILL_AREA(#50911) ;
#50911=FILL_AREA_STYLE('Steel - Satin',(#50918)) ;
#50918=FILL_AREA_STYLE_COLOUR('Steel - Satin',#50925) ;
#50925=COLOUR_RGB('Steel - Satin', 0.31764706, 0.68627451, 0.89019608) ;
ENDSEC;
END-ISO-10303-21;
